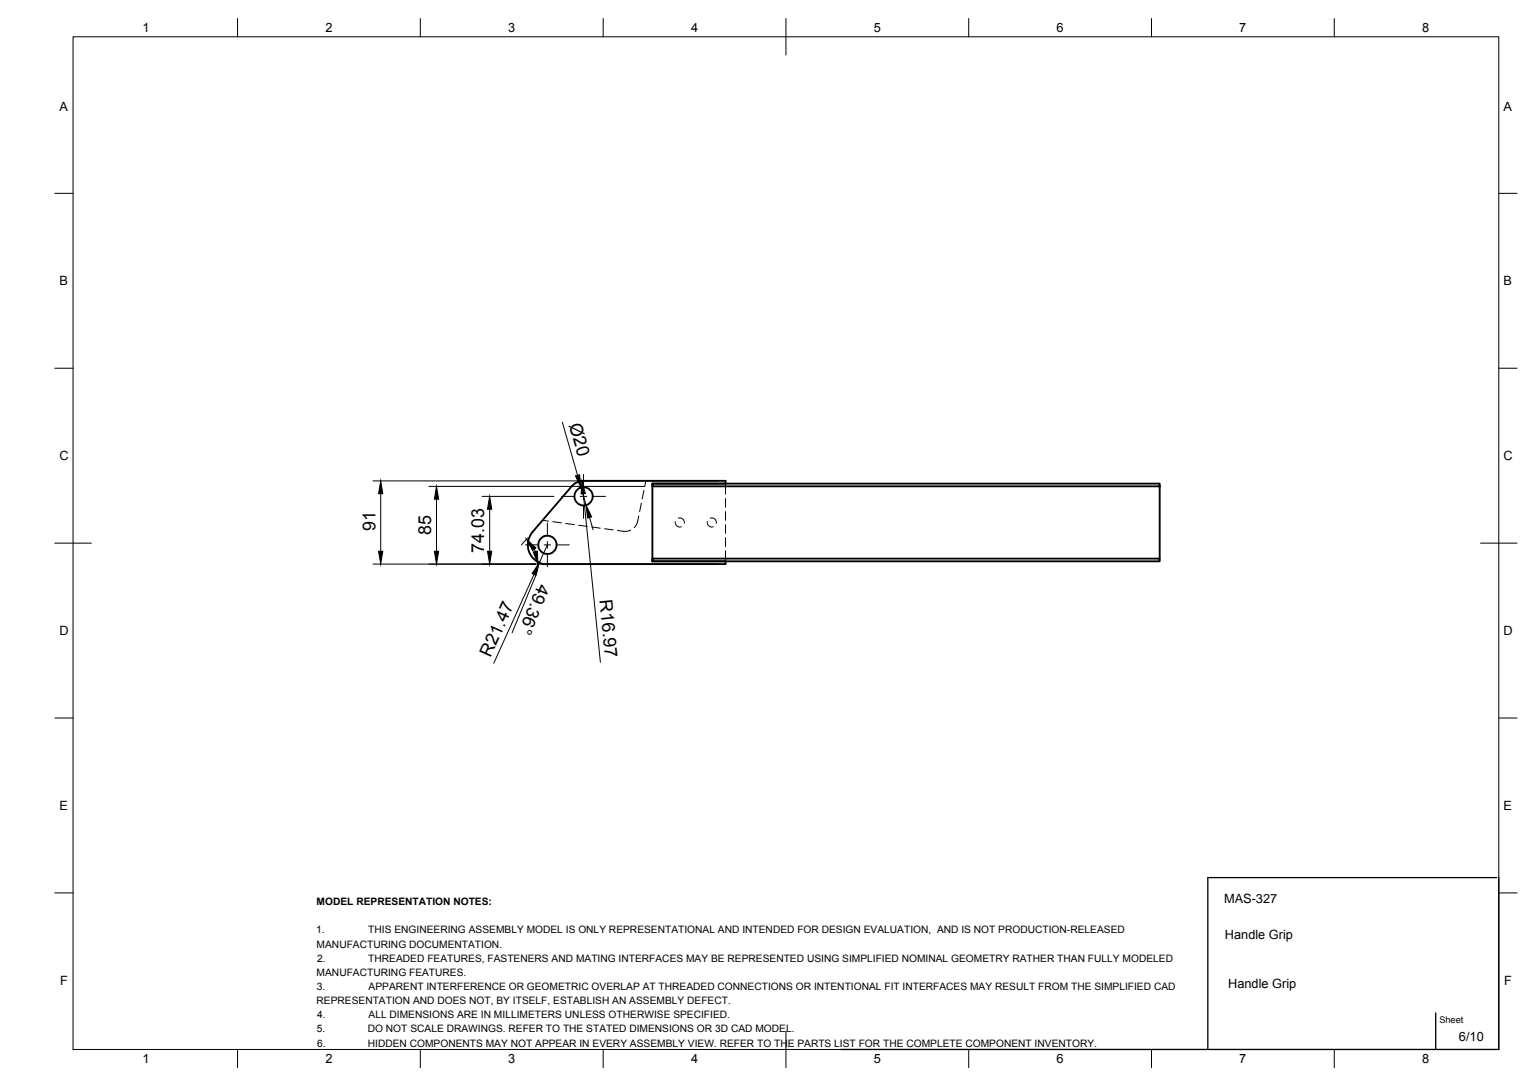
ISO-10303-21;
HEADER;
FILE_DESCRIPTION (('STEP AP214'),
    '1' );
FILE_NAME ('Handle Grip.step',
    '2026-10-06T22:16:42',
    ( '' ),
    ( '' ),
    'SwSTEP 2.0',
    'SolidWorks 2025',
    '' );
FILE_SCHEMA (( 'AUTOMOTIVE_DESIGN' ));
ENDSEC;

DATA;
#6=FILL_AREA_STYLE_COLOUR ( '', #17600 ) ;
#21=CARTESIAN_POINT ( 'NONE',  ( 157.5268905834513475, 193.0332408774651185, -5.999999999999950262 ) ) ;
#34=DIRECTION ( 'NONE',  ( 0.4874675571821265319, 0.8731411001063289490, -0.000000000000000000 ) ) ;
#90=LINE ( 'NONE', #6822, #7245 ) ;
#117=SURFACE_STYLE_FILL_AREA ( #8505 ) ;
#120=VERTEX_POINT ( 'NONE', #20084 ) ;
#156=CARTESIAN_POINT ( 'NONE',  ( 131.8222645499857322, 267.5435007770734046, -19.99999999999997868 ) ) ;
#159=CARTESIAN_POINT ( 'NONE',  ( 138.4260920561042667, 141.9264758756783351, 4.000000000000021316 ) ) ;
#165=CIRCLE ( 'NONE', #18804, 10.00000000000000888 ) ;
#169=ORIENTED_EDGE ( 'NONE', *, *, #12306, .F. ) ;
#196=AXIS2_PLACEMENT_3D ( 'NONE', #10385, #15763, #18755 ) ;
#214=CIRCLE ( 'NONE', #196, 21.47274291077713571 ) ;
#241=ADVANCED_FACE ( 'NONE', ( #14877 ), #10156, .F. ) ;
#244=AXIS2_PLACEMENT_3D ( 'NONE', #16241, #7884, #6214 ) ;
#255=VERTEX_POINT ( 'NONE', #6848 ) ;
#264=CARTESIAN_POINT ( 'NONE',  ( 109.8528842077358405, 344.7014318495014322, 4.000000000000003553 ) ) ;
#267=CARTESIAN_POINT ( 'NONE',  ( 109.8528842077358405, 344.7014318495014322, 272.0939500981630204 ) ) ;
#276=VECTOR ( 'NONE', #19328, 1000.000000000000000 ) ;
#283=MANIFOLD_SOLID_BREP ( 'Cut-Extrude11', #13403 ) ;
#304=CARTESIAN_POINT ( 'NONE',  ( 27.25521010731993243, 314.3399865783788414, -19.99999999999996092 ) ) ;
#348=LINE ( 'NONE', #7078, #20330 ) ;
#428=AXIS2_PLACEMENT_3D ( 'NONE', #10499, #19300, #5628 ) ;
#429=VECTOR ( 'NONE', #16565, 1000.000000000000000 ) ;
#443=ORIENTED_EDGE ( 'NONE', *, *, #13738, .F. ) ;
#452=DIRECTION ( 'NONE',  ( 0.000000000000000000, 0.000000000000000000, 1.000000000000000000 ) ) ;
#455=DIRECTION ( 'NONE',  ( 0.000000000000000000, 0.000000000000000000, 1.000000000000000000 ) ) ;
#474=VECTOR ( 'NONE', #11698, 1000.000000000000114 ) ;
#538=DIRECTION ( 'NONE',  ( 0.000000000000000000, 0.000000000000000000, 1.000000000000000000 ) ) ;
#586=ADVANCED_BREP_SHAPE_REPRESENTATION ( '', ( #14581, #283, #12657 ), #11603 ) ;
#604=ORIENTED_EDGE ( 'NONE', *, *, #3541, .T. ) ;
#632=VECTOR ( 'NONE', #4152, 1000.000000000000227 ) ;
#670=CARTESIAN_POINT ( 'NONE',  ( 111.4021762516569964, 137.5714195593754710, -19.99999999999997868 ) ) ;
#686=ORIENTED_EDGE ( 'NONE', *, *, #10694, .T. ) ;
#720=DIRECTION ( 'NONE',  ( 1.000000000000000000, 0.000000000000000000, 0.000000000000000000 ) ) ;
#758=DIRECTION ( 'NONE',  ( 1.000000000000000000, 0.000000000000000000, 0.000000000000000000 ) ) ;
#763=ADVANCED_FACE ( 'NONE', ( #12088 ), #11983, .F. ) ;
#857=( LENGTH_UNIT ( ) NAMED_UNIT ( * ) SI_UNIT ( .MILLI., .METRE. ) );
#899=ORIENTED_EDGE ( 'NONE', *, *, #19930, .T. ) ;
#900=VECTOR ( 'NONE', #10656, 1000.000000000000114 ) ;
#918=ORIENTED_EDGE ( 'NONE', *, *, #19173, .F. ) ;
#932=VECTOR ( 'NONE', #17024, 1000.000000000000227 ) ;
#984=CARTESIAN_POINT ( 'NONE',  ( 96.62434152388762243, 220.7958015105191976, 4.000000000000021316 ) ) ;
#988=EDGE_CURVE ( 'NONE', #1240, #17720, #90, .T. ) ;
#1025=ORIENTED_EDGE ( 'NONE', *, *, #8453, .F. ) ;
#1031=DIRECTION ( 'NONE',  ( -0.000000000000000000, -0.000000000000000000, -1.000000000000000000 ) ) ;
#1069=ADVANCED_FACE ( 'NONE', ( #8909 ), #19146, .F. ) ;
#1077=PLANE ( 'NONE',  #8255 ) ;
#1102=CARTESIAN_POINT ( 'NONE',  ( 109.8528842077358405, 344.7014318495014322, 4.000000000000003553 ) ) ;
#1138=VERTEX_POINT ( 'NONE', #9014 ) ;
#1157=SHAPE_DEFINITION_REPRESENTATION ( #11328, #17468 ) ;
#1165=ORIENTED_EDGE ( 'NONE', *, *, #14487, .T. ) ;
#1173=CARTESIAN_POINT ( 'NONE',  ( -56.84366818088135176, 789.5005544000622422, -3.999999999999996447 ) ) ;
#1239=EDGE_CURVE ( 'NONE', #13557, #19772, #12755, .T. ) ;
#1240=VERTEX_POINT ( 'NONE', #21355 ) ;
#1246=DIRECTION ( 'NONE',  ( -0.3450121214752274734, 0.9385982292947089300, 0.000000000000000000 ) ) ;
#1257=CYLINDRICAL_SURFACE ( 'NONE', #244, 5.000000000000004441 ) ;
#1258=LINE ( 'NONE', #14373, #6793 ) ;
#1303=VERTEX_POINT ( 'NONE', #3051 ) ;
#1312=DIRECTION ( 'NONE',  ( 0.000000000000000000, 0.000000000000000000, 1.000000000000000000 ) ) ;
#1315=DIRECTION ( 'NONE',  ( -0.3450121214752274179, 0.9385982292947088190, -0.000000000000000000 ) ) ;
#1334=VERTEX_POINT ( 'NONE', #19922 ) ;
#1335=ADVANCED_FACE ( 'NONE', ( #16484 ), #1400, .F. ) ;
#1357=ORIENTED_EDGE ( 'NONE', *, *, #19930, .F. ) ;
#1400=CYLINDRICAL_SURFACE ( 'NONE', #21320, 13.99821153497579651 ) ;
#1424=CARTESIAN_POINT ( 'NONE',  ( 147.5268905834513475, 193.0332408774651185, -5.999999999999976019 ) ) ;
#1451=CARTESIAN_POINT ( 'NONE',  ( 111.4021762516569964, 137.5714195593754710, -19.99999999999997868 ) ) ;
#1461=CARTESIAN_POINT ( 'NONE',  ( 77.34521997529867576, 314.8592298662555322, 272.0939500981630204 ) ) ;
#1503=ORIENTED_EDGE ( 'NONE', *, *, #17821, .F. ) ;
#1506=EDGE_CURVE ( 'NONE', #14220, #7040, #17142, .T. ) ;
#1536=FACE_OUTER_BOUND ( 'NONE', #21519, .T. ) ;
#1587=CARTESIAN_POINT ( 'NONE',  ( 24.43941541943582862, 313.3049502139530205, -19.99999999999997868 ) ) ;
#1590=PLANE ( 'NONE',  #20674 ) ;
#1634=EDGE_LOOP ( 'NONE', ( #6697, #6090, #8259, #12227, #10323, #12958 ) ) ;
#1642=ADVANCED_FACE ( 'NONE', ( #8572 ), #13730, .F. ) ;
#1643=CIRCLE ( 'NONE', #19950, 5.000000000000004441 ) ;
#1657=ORIENTED_EDGE ( 'NONE', *, *, #8443, .F. ) ;
#1725=ORIENTED_EDGE ( 'NONE', *, *, #10803, .F. ) ;
#1745=AXIS2_PLACEMENT_3D ( 'NONE', #8370, #15081, #21817 ) ;
#1778=ORIENTED_EDGE ( 'NONE', *, *, #3369, .T. ) ;
#1784=EDGE_CURVE ( 'NONE', #10393, #12279, #9220, .T. ) ;
#1786=DIRECTION ( 'NONE',  ( -0.000000000000000000, -0.000000000000000000, -1.000000000000000000 ) ) ;
#1826=DIRECTION ( 'NONE',  ( 1.000000000000000000, 0.000000000000000000, 0.000000000000000000 ) ) ;
#1838=CARTESIAN_POINT ( 'NONE',  ( 24.43941541943582862, 313.3049502139530205, 4.000000000000003553 ) ) ;
#1878=VERTEX_POINT ( 'NONE', #4903 ) ;
#1894=ORIENTED_EDGE ( 'NONE', *, *, #13085, .F. ) ;
#1917=CARTESIAN_POINT ( 'NONE',  ( 84.42064422693164261, 282.0082918409407284, 272.0939500981630204 ) ) ;
#1941=DIRECTION ( 'NONE',  ( -0.9385982292947088190, -0.3450121214752277510, 0.000000000000000000 ) ) ;
#1999=FACE_OUTER_BOUND ( 'NONE', #9695, .T. ) ;
#2013=ORIENTED_EDGE ( 'NONE', *, *, #20527, .F. ) ;
#2030=DIRECTION ( 'NONE',  ( -0.8510798296367590998, -0.5250363069212118372, 0.000000000000000000 ) ) ;
#2045=VERTEX_POINT ( 'NONE', #159 ) ;
#2047=ADVANCED_FACE ( 'NONE', ( #15478 ), #18460, .F. ) ;
#2048=CARTESIAN_POINT ( 'NONE',  ( 134.6380592378699532, 268.5785371414991687, -3.999999999999996447 ) ) ;
#2065=CYLINDRICAL_SURFACE ( 'NONE', #12749, 10.00000000000000888 ) ;
#2083=DIRECTION ( 'NONE',  ( -0.000000000000000000, -0.000000000000000000, -1.000000000000000000 ) ) ;
#2116=VERTEX_POINT ( 'NONE', #8653 ) ;
#2172=CIRCLE ( 'NONE', #428, 10.00000000000000888 ) ;
#2213=CARTESIAN_POINT ( 'NONE',  ( -136.6255475934131596, 760.1741454933652449, -19.99999999999996092 ) ) ;
#2221=ORIENTED_EDGE ( 'NONE', *, *, #4577, .F. ) ;
#2224=VERTEX_POINT ( 'NONE', #10307 ) ;
#2233=FACE_BOUND ( 'NONE', #12574, .T. ) ;
#2251=LINE ( 'NONE', #3913, #13441 ) ;
#2275=ADVANCED_FACE ( 'NONE', ( #20124 ), #17010, .F. ) ;
#2297=LINE ( 'NONE', #17284, #12378 ) ;
#2305=ORIENTED_EDGE ( 'NONE', *, *, #5717, .T. ) ;
#2349=EDGE_LOOP ( 'NONE', ( #3996, #12011, #2902, #18773, #11925, #10645 ) ) ;
#2356=ORIENTED_EDGE ( 'NONE', *, *, #5717, .F. ) ;
#2393=ORIENTED_EDGE ( 'NONE', *, *, #15930, .T. ) ;
#2399=EDGE_CURVE ( 'NONE', #9454, #17720, #16871, .T. ) ;
#2403=CARTESIAN_POINT ( 'NONE',  ( 0.000000000000000000, 0.000000000000000000, 0.000000000000000000 ) ) ;
#2417=VERTEX_POINT ( 'NONE', #18539 ) ;
#2424=DIRECTION ( 'NONE',  ( 0.9385982292947088190, 0.3450121214752278620, -0.000000000000000000 ) ) ;
#2436=EDGE_LOOP ( 'NONE', ( #12164, #19467, #16101, #7360, #18553, #14229, #20531, #9668 ) ) ;
#2476=EDGE_CURVE ( 'NONE', #1878, #10563, #4648, .T. ) ;
#2520=EDGE_CURVE ( 'NONE', #2224, #7555, #21637, .T. ) ;
#2547=ORIENTED_EDGE ( 'NONE', *, *, #1784, .F. ) ;
#2592=VERTEX_POINT ( 'NONE', #5201 ) ;
#2600=ORIENTED_EDGE ( 'NONE', *, *, #20829, .T. ) ;
#2619=CARTESIAN_POINT ( 'NONE',  ( 109.8528842077358405, 344.7014318495014322, -19.99999999999997868 ) ) ;
#2624=ORIENTED_EDGE ( 'NONE', *, *, #6281, .F. ) ;
#2626=VERTEX_POINT ( 'NONE', #13889 ) ;
#2628=CARTESIAN_POINT ( 'NONE',  ( 108.9927164799167372, 227.3511983043831037, -5.999999999999976019 ) ) ;
#2641=VECTOR ( 'NONE', #14185, 1000.000000000000227 ) ;
#2650=ORIENTED_EDGE ( 'NONE', *, *, #6268, .T. ) ;
#2672=AXIS2_PLACEMENT_3D ( 'NONE', #18216, #12932, #19656 ) ;
#2678=ORIENTED_EDGE ( 'NONE', *, *, #16774, .T. ) ;
#2682=EDGE_CURVE ( 'NONE', #13485, #15661, #214, .T. ) ;
#2686=CARTESIAN_POINT ( 'NONE',  ( 84.42064422693164261, 282.0082918409407284, 4.000000000000003553 ) ) ;
#2687=DIRECTION ( 'NONE',  ( 0.3450121214752276400, -0.9385982292947087080, 0.000000000000000000 ) ) ;
#2703=DIRECTION ( 'NONE',  ( -0.000000000000000000, -0.000000000000000000, 1.000000000000000000 ) ) ;
#2731=DIRECTION ( 'NONE',  ( 0.000000000000000000, 0.000000000000000000, 1.000000000000000000 ) ) ;
#2770=SURFACE_SIDE_STYLE ('',( #17858 ) ) ;
#2779=LINE ( 'NONE', #21415, #3675 ) ;
#2793=ORIENTED_EDGE ( 'NONE', *, *, #13155, .T. ) ;
#2794=CARTESIAN_POINT ( 'NONE',  ( 121.4021762516569964, 137.5714195593754710, 272.0939500981630204 ) ) ;
#2797=CARTESIAN_POINT ( 'NONE',  ( -136.6255475934131596, 760.1741454933652449, -19.99999999999996092 ) ) ;
#2828=DIRECTION ( 'NONE',  ( 1.000000000000000000, 0.000000000000000000, 0.000000000000000000 ) ) ;
#2831=DIRECTION ( 'NONE',  ( 1.000000000000000000, 0.000000000000000000, -1.723963091245776585E-16 ) ) ;
#2857=PLANE ( 'NONE',  #8341 ) ;
#2861=LINE ( 'NONE', #6061, #16612 ) ;
#2875=ADVANCED_FACE ( 'NONE', ( #11445 ), #11665, .F. ) ;
#2891=DIRECTION ( 'NONE',  ( -0.3450121214752278065, 0.9385982292947087080, -0.000000000000000000 ) ) ;
#2902=ORIENTED_EDGE ( 'NONE', *, *, #10237, .T. ) ;
#2904=LINE ( 'NONE', #16229, #19073 ) ;
#2945=EDGE_CURVE ( 'NONE', #7555, #1878, #9921, .T. ) ;
#2976=ORIENTED_EDGE ( 'NONE', *, *, #9209, .F. ) ;
#2987=ORIENTED_EDGE ( 'NONE', *, *, #15449, .T. ) ;
#2995=ADVANCED_FACE ( 'NONE', ( #14969 ), #21608, .F. ) ;
#2998=ADVANCED_FACE ( 'NONE', ( #1536 ), #13334, .F. ) ;
#3003=ORIENTED_EDGE ( 'NONE', *, *, #988, .F. ) ;
#3010=FACE_OUTER_BOUND ( 'NONE', #8960, .T. ) ;
#3011=PLANE ( 'NONE',  #9235 ) ;
#3051=CARTESIAN_POINT ( 'NONE',  ( 134.6380592378700101, 268.5785371414991687, -3.999999999999996447 ) ) ;
#3078=CARTESIAN_POINT ( 'NONE',  ( 111.4021762516569964, 137.5714195593754710, 272.0939500981630204 ) ) ;
#3126=EDGE_LOOP ( 'NONE', ( #4259, #8088, #5351, #15639 ) ) ;
#3135=DIRECTION ( 'NONE',  ( -0.9385982292947087080, -0.3450121214752278620, 0.000000000000000000 ) ) ;
#3154=ORIENTED_EDGE ( 'NONE', *, *, #5582, .F. ) ;
#3180=CARTESIAN_POINT ( 'NONE',  ( 96.62434152388763664, 220.7958015105191976, -5.999999999999976019 ) ) ;
#3233=VECTOR ( 'NONE', #34, 999.9999999999998863 ) ;
#3333=CIRCLE ( 'NONE', #20241, 10.00000000000000888 ) ;
#3336=DIRECTION ( 'NONE',  ( -0.4874675571821265319, -0.8731411001063289490, 0.000000000000000000 ) ) ;
#3355=ADVANCED_FACE ( 'NONE', ( #3010 ), #5985, .T. ) ;
#3358=CARTESIAN_POINT ( 'NONE',  ( 162.3411339277076308, 184.7625696037766261, 272.0939500981630204 ) ) ;
#3369=EDGE_CURVE ( 'NONE', #13485, #120, #16125, .T. ) ;
#3394=LINE ( 'NONE', #14169, #19787 ) ;
#3400=EDGE_CURVE ( 'NONE', #9553, #2626, #9376, .T. ) ;
#3475=CARTESIAN_POINT ( 'NONE',  ( 139.9279279298906147, 262.8829071470229906, 4.000000000000021316 ) ) ;
#3484=LINE ( 'NONE', #12162, #3741 ) ;
#3486=DIRECTION ( 'NONE',  ( 0.000000000000000000, 0.000000000000000000, 1.000000000000000000 ) ) ;
#3496=VECTOR ( 'NONE', #14530, 1000.000000000000000 ) ;
#3541=EDGE_CURVE ( 'NONE', #9751, #9805, #11486, .T. ) ;
#3590=CARTESIAN_POINT ( 'NONE',  ( -56.84366818088135176, 789.5005544000622422, -19.99999999999997868 ) ) ;
#3603=AXIS2_PLACEMENT_3D ( 'NONE', #9604, #13419, #11757 ) ;
#3617=LINE ( 'NONE', #304, #10490 ) ;
#3659=CARTESIAN_POINT ( 'NONE',  ( 134.6380592378700101, 268.5785371414991687, -19.99999999999997868 ) ) ;
#3675=VECTOR ( 'NONE', #19317, 1000.000000000000227 ) ;
#3680=EDGE_CURVE ( 'NONE', #17077, #17427, #12985, .T. ) ;
#3694=CARTESIAN_POINT ( 'NONE',  ( -136.6255475934131596, 760.1741454933652449, -3.999999999999980904 ) ) ;
#3704=FACE_OUTER_BOUND ( 'NONE', #19461, .T. ) ;
#3718=DIRECTION ( 'NONE',  ( -1.000000000000000000, 0.000000000000000000, 0.000000000000000000 ) ) ;
#3741=VECTOR ( 'NONE', #20560, 1000.000000000000000 ) ;
#3749=DIRECTION ( 'NONE',  ( -1.000000000000000000, 0.000000000000000000, 0.000000000000000000 ) ) ;
#3751=CARTESIAN_POINT ( 'NONE',  ( 84.42064422693164261, 282.0082918409407284, 272.0939500981630204 ) ) ;
#3766=CARTESIAN_POINT ( 'NONE',  ( 138.4260920561042667, 141.9264758756783351, -5.999999999999976019 ) ) ;
#3774=VECTOR ( 'NONE', #8378, 1000.000000000000000 ) ;
#3822=CARTESIAN_POINT ( 'NONE',  ( 131.8222645499855901, 267.5435007770738025, -6.999999999999995559 ) ) ;
#3835=EDGE_CURVE ( 'NONE', #11879, #1138, #3617, .T. ) ;
#3894=DIRECTION ( 'NONE',  ( 0.000000000000000000, 0.000000000000000000, 1.000000000000000000 ) ) ;
#3900=CARTESIAN_POINT ( 'NONE',  ( -56.84366818088135176, 789.5005544000622422, -19.99999999999997868 ) ) ;
#3913=CARTESIAN_POINT ( 'NONE',  ( -133.8097529055291943, 761.2091818577913500, -45.62971374797768220 ) ) ;
#3925=CARTESIAN_POINT ( 'NONE',  ( 162.3411339277076308, 184.7625696037766261, -19.99999999999997868 ) ) ;
#3933=ORIENTED_EDGE ( 'NONE', *, *, #13644, .T. ) ;
#3940=VECTOR ( 'NONE', #21428, 1000.000000000000227 ) ;
#3954=CIRCLE ( 'NONE', #12396, 5.000000000000004441 ) ;
#3986=DIRECTION ( 'NONE',  ( 1.723963091245776585E-16, 6.336983651701954299E-17, 1.000000000000000000 ) ) ;
#3996=ORIENTED_EDGE ( 'NONE', *, *, #11008, .T. ) ;
#4015=EDGE_LOOP ( 'NONE', ( #11908, #16204 ) ) ;
#4028=VECTOR ( 'NONE', #18971, 1000.000000000000000 ) ;
#4077=APPLICATION_CONTEXT ( 'automotive_design' ) ;
#4085=VECTOR ( 'NONE', #8189, 1000.000000000000114 ) ;
#4149=EDGE_CURVE ( 'NONE', #18306, #21732, #21020, .T. ) ;
#4152=DIRECTION ( 'NONE',  ( -0.9385982292947088190, -0.3450121214752274179, 2.040824802394967185E-16 ) ) ;
#4160=FACE_BOUND ( 'NONE', #14959, .T. ) ;
#4177=CARTESIAN_POINT ( 'NONE',  ( 134.6380592378700101, 268.5785371414991687, -19.99999999999997868 ) ) ;
#4227=EDGE_LOOP ( 'NONE', ( #4362, #2305, #1725, #918 ) ) ;
#4237=CARTESIAN_POINT ( 'NONE',  ( 139.9279279298906147, 262.8829071470229906, -5.999999999999976019 ) ) ;
#4259=ORIENTED_EDGE ( 'NONE', *, *, #4577, .T. ) ;
#4313=FACE_BOUND ( 'NONE', #6310, .T. ) ;
#4362=ORIENTED_EDGE ( 'NONE', *, *, #4637, .T. ) ;
#4382=EDGE_CURVE ( 'NONE', #1334, #1240, #7899, .T. ) ;
#4408=EDGE_CURVE ( 'NONE', #10633, #13533, #16149, .T. ) ;
#4413=FILL_AREA_STYLE ('',( #19520 ) ) ;
#4416=LINE ( 'NONE', #13242, #10438 ) ;
#4431=AXIS2_PLACEMENT_3D ( 'NONE', #19436, #1246, #11054 ) ;
#4434=VECTOR ( 'NONE', #16810, 1000.000000000000114 ) ;
#4495=DIRECTION ( 'NONE',  ( 1.723963091245776585E-16, 6.336983651701954299E-17, 1.000000000000000000 ) ) ;
#4527=( NAMED_UNIT ( * ) PLANE_ANGLE_UNIT ( ) SI_UNIT ( $, .RADIAN. ) );
#4561=DIRECTION ( 'NONE',  ( 1.000000000000000000, 0.000000000000000000, 0.000000000000000000 ) ) ;
#4577=EDGE_CURVE ( 'NONE', #17533, #10563, #8559, .T. ) ;
#4589=( NAMED_UNIT ( * ) PLANE_ANGLE_UNIT ( ) SI_UNIT ( $, .RADIAN. ) );
#4617=CARTESIAN_POINT ( 'NONE',  ( 54.85617982533816672, 239.2521282348021714, -19.99999999999996092 ) ) ;
#4618=FACE_OUTER_BOUND ( 'NONE', #16919, .T. ) ;
#4637=EDGE_CURVE ( 'NONE', #9746, #9069, #4827, .T. ) ;
#4648=LINE ( 'NONE', #11367, #4085 ) ;
#4653=CARTESIAN_POINT ( 'NONE',  ( 96.62434152388763664, 220.7958015105191976, 4.000000000000021316 ) ) ;
#4656=( GEOMETRIC_REPRESENTATION_CONTEXT ( 3 ) GLOBAL_UNCERTAINTY_ASSIGNED_CONTEXT ( ( #17219 ) ) GLOBAL_UNIT_ASSIGNED_CONTEXT ( ( #19634, #4527, #9617 ) ) REPRESENTATION_CONTEXT ( 'NONE', 'WORKASPACE' ) );
#4665=CARTESIAN_POINT ( 'NONE',  ( 93.25569916848381524, 126.0916958004080755, -19.99999999999997868 ) ) ;
#4668=ADVANCED_FACE ( 'NONE', ( #13609 ), #20347, .F. ) ;
#4692=ORIENTED_EDGE ( 'NONE', *, *, #4769, .T. ) ;
#4725=DIRECTION ( 'NONE',  ( -1.723963091245776092E-16, -6.336983651701951834E-17, -1.000000000000000000 ) ) ;
#4769=EDGE_CURVE ( 'NONE', #1878, #255, #12607, .T. ) ;
#4773=VECTOR ( 'NONE', #1786, 1000.000000000000000 ) ;
#4775=VERTEX_POINT ( 'NONE', #9307 ) ;
#4780=VECTOR ( 'NONE', #18040, 1000.000000000000000 ) ;
#4827=CIRCLE ( 'NONE', #16087, 10.00000000000000888 ) ;
#4839=LINE ( 'NONE', #16404, #18906 ) ;
#4862=VERTEX_POINT ( 'NONE', #13708 ) ;
#4902=CARTESIAN_POINT ( 'NONE',  ( 27.25521010731993243, 314.3399865783788414, -19.99999999999996092 ) ) ;
#4903=CARTESIAN_POINT ( 'NONE',  ( 134.6380592378699532, 268.5785371414991687, -19.99999999999997868 ) ) ;
#4913=ORIENTED_EDGE ( 'NONE', *, *, #6688, .F. ) ;
#4922=AXIS2_PLACEMENT_3D ( 'NONE', #10433, #10650, #19233 ) ;
#4959=CARTESIAN_POINT ( 'NONE',  ( 137.5268905834513191, 193.0332408774651185, 272.0939500981630204 ) ) ;
#5018=DIRECTION ( 'NONE',  ( -0.9385982292947088190, -0.3450121214752277510, 0.000000000000000000 ) ) ;
#5027=CARTESIAN_POINT ( 'NONE',  ( 107.0370895198517189, 343.6663954850758955, -19.99999999999997868 ) ) ;
#5046=PLANE ( 'NONE',  #3603 ) ;
#5057=ORIENTED_EDGE ( 'NONE', *, *, #13409, .T. ) ;
#5066=DIRECTION ( 'NONE',  ( -0.000000000000000000, -0.000000000000000000, -1.000000000000000000 ) ) ;
#5107=CARTESIAN_POINT ( 'NONE',  ( -56.84366818088135176, 789.5005544000622422, -3.999999999999996447 ) ) ;
#5138=VERTEX_POINT ( 'NONE', #7655 ) ;
#5143=CARTESIAN_POINT ( 'NONE',  ( 24.43941541943582862, 313.3049502139530205, 4.000000000000003553 ) ) ;
#5157=DIRECTION ( 'NONE',  ( -0.3450121214752276955, 0.9385982292947087080, -0.000000000000000000 ) ) ;
#5177=EDGE_CURVE ( 'NONE', #20168, #2045, #17869, .T. ) ;
#5188=AXIS2_PLACEMENT_3D ( 'NONE', #9596, #16187, #12564 ) ;
#5201=CARTESIAN_POINT ( 'NONE',  ( -136.6255475934131596, 760.1741454933652449, -3.999999999999980904 ) ) ;
#5223=ORIENTED_EDGE ( 'NONE', *, *, #17821, .T. ) ;
#5255=LINE ( 'NONE', #5566, #8719 ) ;
#5292=SURFACE_STYLE_USAGE ( .BOTH. , #18633 ) ;
#5294=EDGE_CURVE ( 'NONE', #2224, #1138, #12811, .T. ) ;
#5299=ORIENTED_EDGE ( 'NONE', *, *, #4637, .F. ) ;
#5314=FACE_OUTER_BOUND ( 'NONE', #21176, .T. ) ;
#5351=ORIENTED_EDGE ( 'NONE', *, *, #2945, .F. ) ;
#5356=CARTESIAN_POINT ( 'NONE',  ( 24.43941541943582862, 313.3049502139530205, -19.99999999999997868 ) ) ;
#5368=EDGE_CURVE ( 'NONE', #16231, #17982, #15120, .T. ) ;
#5387=LINE ( 'NONE', #10360, #15011 ) ;
#5445=DIRECTION ( 'NONE',  ( 0.3450121214752278065, -0.9385982292947087080, -0.000000000000000000 ) ) ;
#5566=CARTESIAN_POINT ( 'NONE',  ( -56.84366818088135176, 789.5005544000622422, -3.999999999999996447 ) ) ;
#5574=VERTEX_POINT ( 'NONE', #19191 ) ;
#5582=EDGE_CURVE ( 'NONE', #13398, #4862, #20344, .T. ) ;
#5628=DIRECTION ( 'NONE',  ( 1.000000000000000000, 0.000000000000000000, 0.000000000000000000 ) ) ;
#5632=ORIENTED_EDGE ( 'NONE', *, *, #6281, .T. ) ;
#5634=AXIS2_PLACEMENT_3D ( 'NONE', #3751, #12113, #15102 ) ;
#5684=ADVANCED_FACE ( 'NONE', ( #14543 ), #5046, .F. ) ;
#5700=PLANE ( 'NONE',  #21103 ) ;
#5717=EDGE_CURVE ( 'NONE', #9069, #5138, #2861, .T. ) ;
#5736=DIRECTION ( 'NONE',  ( 1.000000000000000000, 0.000000000000000000, -1.734723475976805615E-16 ) ) ;
#5801=AXIS2_PLACEMENT_3D ( 'NONE', #20467, #18807, #10442 ) ;
#5841=DIRECTION ( 'NONE',  ( 1.000000000000000000, 0.000000000000000000, -1.734723475976805615E-16 ) ) ;
#5856=VECTOR ( 'NONE', #16236, 1000.000000000000227 ) ;
#5875=EDGE_LOOP ( 'NONE', ( #15537, #17424, #3154, #11551 ) ) ;
#5910=ORIENTED_EDGE ( 'NONE', *, *, #20563, .T. ) ;
#5945=AXIS2_PLACEMENT_3D ( 'NONE', #2628, #13908, #15568 ) ;
#5953=ADVANCED_FACE ( 'NONE', ( #7031 ), #2065, .F. ) ;
#5960=EDGE_CURVE ( 'NONE', #10863, #7143, #3394, .T. ) ;
#5985=PLANE ( 'NONE',  #4431 ) ;
#6018=CARTESIAN_POINT ( 'NONE',  ( 107.0370895198517189, 343.6663954850758955, -3.999999999999996447 ) ) ;
#6034=APPLICATION_CONTEXT ( 'automotive_design' ) ;
#6039=VECTOR ( 'NONE', #15498, 1000.000000000000227 ) ;
#6048=AXIS2_PLACEMENT_3D ( 'NONE', #18233, #13494, #3135 ) ;
#6061=CARTESIAN_POINT ( 'NONE',  ( 157.5268905834513475, 193.0332408774651185, 272.0939500981630204 ) ) ;
#6075=ORIENTED_EDGE ( 'NONE', *, *, #17476, .T. ) ;
#6085=ORIENTED_EDGE ( 'NONE', *, *, #10169, .F. ) ;
#6090=ORIENTED_EDGE ( 'NONE', *, *, #4408, .F. ) ;
#6140=CARTESIAN_POINT ( 'NONE',  ( 138.4260920561042667, 141.9264758756783351, -5.999999999999976019 ) ) ;
#6214=DIRECTION ( 'NONE',  ( -1.000000000000000000, 0.000000000000000000, 0.000000000000000000 ) ) ;
#6254=DIRECTION ( 'NONE',  ( 0.4874675571821264763, 0.8731411001063288380, 0.000000000000000000 ) ) ;
#6255=LINE ( 'NONE', #17714, #19428 ) ;
#6268=EDGE_CURVE ( 'NONE', #17720, #10563, #10329, .T. ) ;
#6274=CYLINDRICAL_SURFACE ( 'NONE', #9672, 16.96660865288809816 ) ;
#6281=EDGE_CURVE ( 'NONE', #8122, #12991, #10294, .T. ) ;
#6310=EDGE_LOOP ( 'NONE', ( #2393, #604 ) ) ;
#6320=VERTEX_POINT ( 'NONE', #5143 ) ;
#6347=ORIENTED_EDGE ( 'NONE', *, *, #2520, .F. ) ;
#6383=CARTESIAN_POINT ( 'NONE',  ( -136.6255475934131596, 760.1741454933652449, -3.999999999999980904 ) ) ;
#6384=LINE ( 'NONE', #4617, #15109 ) ;
#6401=ORIENTED_EDGE ( 'NONE', *, *, #2476, .T. ) ;
#6419=PRODUCT ( 'Handle Grip', 'Handle Grip', '', ( #19556 ) ) ;
#6420=COLOUR_RGB ( '', 0.72549020, 0.75294118, 0.79215686) ;
#6454=DIRECTION ( 'NONE',  ( -0.000000000000000000, -0.000000000000000000, -1.000000000000000000 ) ) ;
#6485=ORIENTED_EDGE ( 'NONE', *, *, #3835, .T. ) ;
#6545=AXIS2_PLACEMENT_3D ( 'NONE', #267, #5018, #8439 ) ;
#6548=EDGE_LOOP ( 'NONE', ( #17582, #11767, #6991, #9856 ) ) ;
#6556=VECTOR ( 'NONE', #5445, 1000.000000000000114 ) ;
#6601=CARTESIAN_POINT ( 'NONE',  ( 72.34521997529867576, 314.8592298662555322, 272.0939500981630204 ) ) ;
#6603=ORIENTED_EDGE ( 'NONE', *, *, #13085, .T. ) ;
#6610=AXIS2_PLACEMENT_3D ( 'NONE', #14704, #14590, #21667 ) ;
#6634=AXIS2_PLACEMENT_3D ( 'NONE', #4237, #21003, #8892 ) ;
#6655=PRODUCT_DEFINITION_CONTEXT ( 'detailed design', #4077, 'design' ) ;
#6688=EDGE_CURVE ( 'NONE', #6320, #13485, #1258, .T. ) ;
#6697=ORIENTED_EDGE ( 'NONE', *, *, #18056, .F. ) ;
#6743=ORIENTED_EDGE ( 'NONE', *, *, #7316, .F. ) ;
#6761=CARTESIAN_POINT ( 'NONE',  ( 54.85617982533818804, 239.2521282348021714, -19.99999999999996092 ) ) ;
#6782=CARTESIAN_POINT ( 'NONE',  ( 93.25569916848381524, 126.0916958004080755, 272.0939500981630204 ) ) ;
#6793=VECTOR ( 'NONE', #2687, 1000.000000000000227 ) ;
#6814=CARTESIAN_POINT ( 'NONE',  ( -133.8097529055291943, 761.2091818577913500, -6.999999999999982236 ) ) ;
#6822=CARTESIAN_POINT ( 'NONE',  ( 109.8528842077358405, 344.7014318495014322, -19.99999999999997868 ) ) ;
#6838=DIRECTION ( 'NONE',  ( 0.000000000000000000, 0.000000000000000000, 1.000000000000000000 ) ) ;
#6848=CARTESIAN_POINT ( 'NONE',  ( 54.85617982533816672, 239.2521282348021714, -19.99999999999996092 ) ) ;
#6884=VECTOR ( 'NONE', #10224, 1000.000000000000227 ) ;
#6904=DIRECTION ( 'NONE',  ( -0.3450121214752274179, 0.9385982292947088190, -7.395570986446985676E-32 ) ) ;
#6913=DIRECTION ( 'NONE',  ( 1.000000000000000000, 0.000000000000000000, 0.000000000000000000 ) ) ;
#6931=VECTOR ( 'NONE', #7320, 1000.000000000000000 ) ;
#6991=ORIENTED_EDGE ( 'NONE', *, *, #8037, .T. ) ;
#7018=VERTEX_POINT ( 'NONE', #11836 ) ;
#7031=FACE_OUTER_BOUND ( 'NONE', #4227, .T. ) ;
#7040=VERTEX_POINT ( 'NONE', #15256 ) ;
#7050=DIRECTION ( 'NONE',  ( 0.000000000000000000, 0.000000000000000000, 1.000000000000000000 ) ) ;
#7062=( NAMED_UNIT ( * ) SI_UNIT ( $, .STERADIAN. ) SOLID_ANGLE_UNIT ( ) );
#7078=CARTESIAN_POINT ( 'NONE',  ( 24.43941541943582862, 313.3049502139530205, 272.0939500981630204 ) ) ;
#7084=CARTESIAN_POINT ( 'NONE',  ( 162.3411339277076308, 184.7625696037766261, 272.0939500981630204 ) ) ;
#7097=ORIENTED_EDGE ( 'NONE', *, *, #20930, .T. ) ;
#7100=DIRECTION ( 'NONE',  ( 0.9385982292947088190, 0.3450121214752276955, -0.000000000000000000 ) ) ;
#7143=VERTEX_POINT ( 'NONE', #21664 ) ;
#7144=DIRECTION ( 'NONE',  ( 0.000000000000000000, 0.000000000000000000, 1.000000000000000000 ) ) ;
#7149=ORIENTED_EDGE ( 'NONE', *, *, #19173, .T. ) ;
#7169=DIRECTION ( 'NONE',  ( -0.9385982292947088190, -0.3450121214752274179, 2.040824802394967185E-16 ) ) ;
#7234=ORIENTED_EDGE ( 'NONE', *, *, #21469, .F. ) ;
#7245=VECTOR ( 'NONE', #5157, 1000.000000000000227 ) ;
#7279=AXIS2_PLACEMENT_3D ( 'NONE', #21086, #8862, #14019 ) ;
#7291=VECTOR ( 'NONE', #1941, 999.9999999999998863 ) ;
#7298=DIRECTION ( 'NONE',  ( -0.3450121214752275844, 0.9385982292947088190, 0.000000000000000000 ) ) ;
#7316=EDGE_CURVE ( 'NONE', #255, #11879, #6384, .T. ) ;
#7320=DIRECTION ( 'NONE',  ( 0.000000000000000000, 0.000000000000000000, -1.000000000000000000 ) ) ;
#7330=ORIENTED_EDGE ( 'NONE', *, *, #20404, .F. ) ;
#7360=ORIENTED_EDGE ( 'NONE', *, *, #20527, .T. ) ;
#7403=DIRECTION ( 'NONE',  ( -0.3450121214752278065, 0.9385982292947087080, 0.000000000000000000 ) ) ;
#7411=ORIENTED_EDGE ( 'NONE', *, *, #20563, .F. ) ;
#7420=ORIENTED_EDGE ( 'NONE', *, *, #2520, .T. ) ;
#7444=ORIENTED_EDGE ( 'NONE', *, *, #15000, .T. ) ;
#7463=EDGE_LOOP ( 'NONE', ( #6485, #8526, #443, #18927 ) ) ;
#7473=EDGE_LOOP ( 'NONE', ( #8482, #10075, #9524, #20401 ) ) ;
#7483=CARTESIAN_POINT ( 'NONE',  ( 57.67197451322198276, 240.2871645992281628, -6.999999999999982236 ) ) ;
#7519=EDGE_LOOP ( 'NONE', ( #4692, #16423, #7420, #12447 ) ) ;
#7555=VERTEX_POINT ( 'NONE', #8822 ) ;
#7621=VECTOR ( 'NONE', #1031, 1000.000000000000000 ) ;
#7644=EDGE_CURVE ( 'NONE', #9069, #9746, #3333, .T. ) ;
#7655=CARTESIAN_POINT ( 'NONE',  ( 157.5268905834513475, 193.0332408774651185, -19.99999999999997868 ) ) ;
#7706=DIRECTION ( 'NONE',  ( 1.723963091245776585E-16, 6.336983651701954299E-17, 1.000000000000000000 ) ) ;
#7773=ORIENTED_EDGE ( 'NONE', *, *, #8895, .F. ) ;
#7775=CARTESIAN_POINT ( 'NONE',  ( -136.6255475934131596, 760.1741454933652449, -3.999999999999980904 ) ) ;
#7824=ORIENTED_EDGE ( 'NONE', *, *, #10237, .F. ) ;
#7826=LINE ( 'NONE', #16396, #3496 ) ;
#7850=EDGE_CURVE ( 'NONE', #19966, #4862, #18268, .T. ) ;
#7882=LINE ( 'NONE', #7775, #5856 ) ;
#7884=DIRECTION ( 'NONE',  ( -0.000000000000000000, -0.000000000000000000, -1.000000000000000000 ) ) ;
#7888=CYLINDRICAL_SURFACE ( 'NONE', #6610, 21.47274291077713571 ) ;
#7899=LINE ( 'NONE', #12846, #17502 ) ;
#7914=DIRECTION ( 'NONE',  ( -0.000000000000000000, -0.000000000000000000, 1.000000000000000000 ) ) ;
#8037=EDGE_CURVE ( 'NONE', #8122, #21618, #11078, .T. ) ;
#8047=DIRECTION ( 'NONE',  ( 1.000000000000000000, 0.000000000000000000, 0.000000000000000000 ) ) ;
#8067=ORIENTED_EDGE ( 'NONE', *, *, #9771, .F. ) ;
#8088=ORIENTED_EDGE ( 'NONE', *, *, #2476, .F. ) ;
#8122=VERTEX_POINT ( 'NONE', #19460 ) ;
#8176=VERTEX_POINT ( 'NONE', #14171 ) ;
#8189=DIRECTION ( 'NONE',  ( -0.3450121214752278065, 0.9385982292947087080, -0.000000000000000000 ) ) ;
#8193=DIRECTION ( 'NONE',  ( 0.4683024526015100442, -0.8835682276357669229, 0.000000000000000000 ) ) ;
#8226=ORIENTED_EDGE ( 'NONE', *, *, #17669, .F. ) ;
#8255=AXIS2_PLACEMENT_3D ( 'NONE', #16276, #7706, #2831 ) ;
#8257=ADVANCED_FACE ( 'NONE', ( #14714 ), #15043, .F. ) ;
#8259=ORIENTED_EDGE ( 'NONE', *, *, #11008, .F. ) ;
#8287=ORIENTED_EDGE ( 'NONE', *, *, #9209, .T. ) ;
#8318=DIRECTION ( 'NONE',  ( -0.9385982292947087080, -0.3450121214752276955, -0.000000000000000000 ) ) ;
#8323=FACE_OUTER_BOUND ( 'NONE', #7519, .T. ) ;
#8341=AXIS2_PLACEMENT_3D ( 'NONE', #10816, #21167, #15973 ) ;
#8370=CARTESIAN_POINT ( 'NONE',  ( 72.34521997529867576, 314.8592298662555322, -4.000000000000003553 ) ) ;
#8378=DIRECTION ( 'NONE',  ( 0.000000000000000000, 0.000000000000000000, -1.000000000000000000 ) ) ;
#8393=CIRCLE ( 'NONE', #21765, 21.47274291077713571 ) ;
#8437=CARTESIAN_POINT ( 'NONE',  ( 162.3411339277076308, 184.7625696037766261, -19.99999999999997868 ) ) ;
#8439=DIRECTION ( 'NONE',  ( 0.3450121214752276955, -0.9385982292947087080, 0.000000000000000000 ) ) ;
#8443=EDGE_CURVE ( 'NONE', #2592, #20087, #9876, .T. ) ;
#8444=VECTOR ( 'NONE', #14827, 1000.000000000000000 ) ;
#8453=EDGE_CURVE ( 'NONE', #15661, #10393, #3484, .T. ) ;
#8482=ORIENTED_EDGE ( 'NONE', *, *, #14487, .F. ) ;
#8505=FILL_AREA_STYLE ('',( #6 ) ) ;
#8521=LINE ( 'NONE', #6761, #9991 ) ;
#8526=ORIENTED_EDGE ( 'NONE', *, *, #5294, .F. ) ;
#8552=DIRECTION ( 'NONE',  ( 0.000000000000000000, 0.000000000000000000, -1.000000000000000000 ) ) ;
#8559=LINE ( 'NONE', #5027, #14343 ) ;
#8572=FACE_OUTER_BOUND ( 'NONE', #16584, .T. ) ;
#8620=CIRCLE ( 'NONE', #18104, 13.99821153497579651 ) ;
#8644=PLANE ( 'NONE',  #14648 ) ;
#8653=CARTESIAN_POINT ( 'NONE',  ( 79.42064422693164261, 282.0082918409407284, 4.000000000000003553 ) ) ;
#8667=LINE ( 'NONE', #2048, #4434 ) ;
#8672=AXIS2_PLACEMENT_3D ( 'NONE', #3078, #9814, #20070 ) ;
#8673=CARTESIAN_POINT ( 'NONE',  ( 108.9927164799167372, 227.3511983043831037, -5.999999999999976019 ) ) ;
#8701=CIRCLE ( 'NONE', #5188, 5.000000000000004441 ) ;
#8719=VECTOR ( 'NONE', #19026, 1000.000000000000114 ) ;
#8721=PLANE ( 'NONE',  #13104 ) ;
#8738=CARTESIAN_POINT ( 'NONE',  ( 57.67197451322208934, 240.2871645992278218, 0.000000000000000000 ) ) ;
#8776=ORIENTED_EDGE ( 'NONE', *, *, #8037, .F. ) ;
#8822=CARTESIAN_POINT ( 'NONE',  ( 134.6380592378699532, 268.5785371414991687, -3.999999999999996447 ) ) ;
#8827=( LENGTH_UNIT ( ) NAMED_UNIT ( * ) SI_UNIT ( .MILLI., .METRE. ) );
#8830=EDGE_LOOP ( 'NONE', ( #5910, #16306 ) ) ;
#8858=ORIENTED_EDGE ( 'NONE', *, *, #9429, .F. ) ;
#8862=DIRECTION ( 'NONE',  ( 0.000000000000000000, 0.000000000000000000, 1.000000000000000000 ) ) ;
#8883=ORIENTED_EDGE ( 'NONE', *, *, #13409, .F. ) ;
#8887=EDGE_CURVE ( 'NONE', #7018, #20087, #8521, .T. ) ;
#8892=DIRECTION ( 'NONE',  ( -0.8510798296367592108, -0.5250363069212118372, 0.000000000000000000 ) ) ;
#8895=EDGE_CURVE ( 'NONE', #10633, #10863, #18320, .T. ) ;
#8909=FACE_OUTER_BOUND ( 'NONE', #2436, .T. ) ;
#8945=LINE ( 'NONE', #3766, #4028 ) ;
#8960=EDGE_LOOP ( 'NONE', ( #17910, #9586, #14470, #6603, #3933, #13236, #15986, #20451 ) ) ;
#8966=LINE ( 'NONE', #15672, #6931 ) ;
#8989=EDGE_LOOP ( 'NONE', ( #2624, #12791 ) ) ;
#9014=CARTESIAN_POINT ( 'NONE',  ( 27.25521010731993243, 314.3399865783788414, -3.999999999999980904 ) ) ;
#9039=DIRECTION ( 'NONE',  ( 0.4683024526015100442, -0.8835682276357669229, 0.000000000000000000 ) ) ;
#9069=VERTEX_POINT ( 'NONE', #21 ) ;
#9149=CARTESIAN_POINT ( 'NONE',  ( 107.0370895198517189, 343.6663954850758955, -3.999999999999996447 ) ) ;
#9183=ORIENTED_EDGE ( 'NONE', *, *, #18437, .F. ) ;
#9209=EDGE_CURVE ( 'NONE', #120, #10393, #8393, .T. ) ;
#9220=LINE ( 'NONE', #3925, #900 ) ;
#9235=AXIS2_PLACEMENT_3D ( 'NONE', #5107, #16669, #13482 ) ;
#9241=FACE_BOUND ( 'NONE', #8989, .T. ) ;
#9247=VECTOR ( 'NONE', #8552, 1000.000000000000000 ) ;
#9307=CARTESIAN_POINT ( 'NONE',  ( -136.6255475934131596, 760.1741454933652449, -19.99999999999996092 ) ) ;
#9320=ADVANCED_FACE ( 'NONE', ( #17951 ), #2857, .F. ) ;
#9374=CARTESIAN_POINT ( 'NONE',  ( 134.6380592378699532, 268.5785371414991687, -19.99999999999997868 ) ) ;
#9376=CIRCLE ( 'NONE', #2672, 10.00000000000000888 ) ;
#9378=DIRECTION ( 'NONE',  ( 0.000000000000000000, 0.000000000000000000, 1.000000000000000000 ) ) ;
#9418=CARTESIAN_POINT ( 'NONE',  ( 79.42064422693164261, 282.0082918409407284, 272.0939500981630204 ) ) ;
#9429=EDGE_CURVE ( 'NONE', #2116, #19966, #1643, .T. ) ;
#9431=DIRECTION ( 'NONE',  ( 0.000000000000000000, 0.000000000000000000, 1.000000000000000000 ) ) ;
#9448=EDGE_LOOP ( 'NONE', ( #5632, #2987, #7411, #8776 ) ) ;
#9454=VERTEX_POINT ( 'NONE', #1102 ) ;
#9461=EDGE_CURVE ( 'NONE', #8176, #21618, #14298, .T. ) ;
#9493=DIRECTION ( 'NONE',  ( 1.723963091245776585E-16, 6.336983651701954299E-17, 1.000000000000000000 ) ) ;
#9510=SURFACE_STYLE_USAGE ( .BOTH. , #2770 ) ;
#9524=ORIENTED_EDGE ( 'NONE', *, *, #20404, .T. ) ;
#9532=DIRECTION ( 'NONE',  ( -0.000000000000000000, -0.000000000000000000, -1.000000000000000000 ) ) ;
#9535=DIRECTION ( 'NONE',  ( -0.000000000000000000, -0.000000000000000000, -1.000000000000000000 ) ) ;
#9540=FACE_OUTER_BOUND ( 'NONE', #6548, .T. ) ;
#9553=VERTEX_POINT ( 'NONE', #13220 ) ;
#9576=AXIS2_PLACEMENT_3D ( 'NONE', #7084, #18546, #3336 ) ;
#9578=VECTOR ( 'NONE', #7169, 1000.000000000000227 ) ;
#9586=ORIENTED_EDGE ( 'NONE', *, *, #18437, .T. ) ;
#9596=CARTESIAN_POINT ( 'NONE',  ( 72.34521997529867576, 314.8592298662555322, 4.000000000000003553 ) ) ;
#9599=DIRECTION ( 'NONE',  ( -0.000000000000000000, -0.000000000000000000, -1.000000000000000000 ) ) ;
#9604=CARTESIAN_POINT ( 'NONE',  ( 57.67197451322198276, 240.2871645992281628, -45.62971374797768220 ) ) ;
#9617=( NAMED_UNIT ( * ) SI_UNIT ( $, .STERADIAN. ) SOLID_ANGLE_UNIT ( ) );
#9631=ORIENTED_EDGE ( 'NONE', *, *, #5582, .T. ) ;
#9662=ORIENTED_EDGE ( 'NONE', *, *, #5177, .T. ) ;
#9668=ORIENTED_EDGE ( 'NONE', *, *, #8887, .F. ) ;
#9671=LINE ( 'NONE', #6018, #10541 ) ;
#9672=AXIS2_PLACEMENT_3D ( 'NONE', #19503, #9599, #19396 ) ;
#9695=EDGE_LOOP ( 'NONE', ( #12135, #1657, #8067, #2793 ) ) ;
#9704=CARTESIAN_POINT ( 'NONE',  ( 134.6380592378700101, 268.5785371414991687, -3.999999999999996447 ) ) ;
#9721=ORIENTED_EDGE ( 'NONE', *, *, #13644, .F. ) ;
#9746=VERTEX_POINT ( 'NONE', #19055 ) ;
#9751=VERTEX_POINT ( 'NONE', #13865 ) ;
#9771=EDGE_CURVE ( 'NONE', #4775, #2592, #5387, .T. ) ;
#9773=ORIENTED_EDGE ( 'NONE', *, *, #18784, .F. ) ;
#9805=VERTEX_POINT ( 'NONE', #18948 ) ;
#9814=DIRECTION ( 'NONE',  ( -0.000000000000000000, -0.000000000000000000, -1.000000000000000000 ) ) ;
#9835=AXIS2_PLACEMENT_3D ( 'NONE', #11221, #19827, #21488 ) ;
#9856=ORIENTED_EDGE ( 'NONE', *, *, #9461, .F. ) ;
#9876=LINE ( 'NONE', #3694, #6556 ) ;
#9909=DIRECTION ( 'NONE',  ( 0.4683024526015100442, -0.8835682276357670339, 0.000000000000000000 ) ) ;
#9921=LINE ( 'NONE', #18508, #16407 ) ;
#9944=EDGE_LOOP ( 'NONE', ( #7097, #15565, #6347, #19492 ) ) ;
#9951=DIRECTION ( 'NONE',  ( 0.9385982292947087080, 0.3450121214752278620, -1.836742322155470738E-16 ) ) ;
#9971=ORIENTED_EDGE ( 'NONE', *, *, #18784, .T. ) ;
#9976=DIRECTION ( 'NONE',  ( 1.000000000000000000, 0.000000000000000000, 0.000000000000000000 ) ) ;
#9990=ORIENTED_EDGE ( 'NONE', *, *, #17001, .F. ) ;
#9991=VECTOR ( 'NONE', #11474, 1000.000000000000000 ) ;
#10065=ORIENTED_EDGE ( 'NONE', *, *, #11634, .T. ) ;
#10075=ORIENTED_EDGE ( 'NONE', *, *, #3400, .T. ) ;
#10079=FACE_OUTER_BOUND ( 'NONE', #15669, .T. ) ;
#10129=VECTOR ( 'NONE', #2703, 1000.000000000000000 ) ;
#10131=ORIENTED_EDGE ( 'NONE', *, *, #8453, .T. ) ;
#10133=LINE ( 'NONE', #20377, #21811 ) ;
#10151=AXIS2_PLACEMENT_3D ( 'NONE', #11625, #21450, #16255 ) ;
#10156=CYLINDRICAL_SURFACE ( 'NONE', #5634, 5.000000000000004441 ) ;
#10169=EDGE_CURVE ( 'NONE', #9454, #6320, #17030, .T. ) ;
#10177=ORIENTED_EDGE ( 'NONE', *, *, #11634, .F. ) ;
#10224=DIRECTION ( 'NONE',  ( 0.9385982292947090411, 0.3450121214752271959, -1.756657601269562932E-16 ) ) ;
#10237=EDGE_CURVE ( 'NONE', #10863, #15960, #16110, .T. ) ;
#10287=VECTOR ( 'NONE', #13787, 1000.000000000000000 ) ;
#10294=CIRCLE ( 'NONE', #20143, 5.000000000000004441 ) ;
#10302=STYLED_ITEM ( 'NONE', ( #16207 ), #14581 ) ;
#10307=CARTESIAN_POINT ( 'NONE',  ( 54.85617982533816672, 239.2521282348021714, -3.999999999999980904 ) ) ;
#10318=DIRECTION ( 'NONE',  ( 1.915514545828640458E-16, 7.041092946335503408E-17, 1.000000000000000000 ) ) ;
#10322=LINE ( 'NONE', #13721, #932 ) ;
#10323=ORIENTED_EDGE ( 'NONE', *, *, #988, .T. ) ;
#10329=LINE ( 'NONE', #5356, #6039 ) ;
#10348=ADVANCED_FACE ( 'NONE', ( #20677 ), #12616, .F. ) ;
#10360=CARTESIAN_POINT ( 'NONE',  ( -136.6255475934131596, 760.1741454933652449, -19.99999999999996092 ) ) ;
#10385=CARTESIAN_POINT ( 'NONE',  ( 111.4021762516569964, 137.5714195593754710, 4.000000000000003553 ) ) ;
#10393=VERTEX_POINT ( 'NONE', #15703 ) ;
#10415=CARTESIAN_POINT ( 'NONE',  ( -59.65946286876558702, 788.4655180356369328, -6.999999999999995559 ) ) ;
#10433=CARTESIAN_POINT ( 'NONE',  ( 147.5268905834513475, 193.0332408774651185, 272.0939500981630204 ) ) ;
#10438=VECTOR ( 'NONE', #19524, 1000.000000000000000 ) ;
#10442=DIRECTION ( 'NONE',  ( 0.9385982292947087080, 0.3450121214752276955, 0.000000000000000000 ) ) ;
#10490=VECTOR ( 'NONE', #7144, 1000.000000000000000 ) ;
#10499=CARTESIAN_POINT ( 'NONE',  ( 111.4021762516569964, 137.5714195593754710, -19.99999999999997868 ) ) ;
#10541=VECTOR ( 'NONE', #21461, 1000.000000000000000 ) ;
#10563=VERTEX_POINT ( 'NONE', #16455 ) ;
#10615=ORIENTED_EDGE ( 'NONE', *, *, #7850, .F. ) ;
#10633=VERTEX_POINT ( 'NONE', #11616 ) ;
#10644=CARTESIAN_POINT ( 'NONE',  ( -133.8097529055291943, 761.2091818577913500, -6.999999999999982236 ) ) ;
#10645=ORIENTED_EDGE ( 'NONE', *, *, #21469, .T. ) ;
#10648=CIRCLE ( 'NONE', #13460, 16.96660865288809816 ) ;
#10650=DIRECTION ( 'NONE',  ( -0.000000000000000000, -0.000000000000000000, -1.000000000000000000 ) ) ;
#10656=DIRECTION ( 'NONE',  ( 0.4874675571821264763, 0.8731411001063288380, -0.000000000000000000 ) ) ;
#10693=ORIENTED_EDGE ( 'NONE', *, *, #4382, .F. ) ;
#10694=EDGE_CURVE ( 'NONE', #19966, #2116, #17834, .T. ) ;
#10695=DIRECTION ( 'NONE',  ( 0.9385982292947089300, 0.3450121214752274734, 0.000000000000000000 ) ) ;
#10696=ORIENTED_EDGE ( 'NONE', *, *, #5177, .F. ) ;
#10722=ADVANCED_FACE ( 'NONE', ( #9540 ), #1257, .F. ) ;
#10744=CARTESIAN_POINT ( 'NONE',  ( 134.6380592378699532, 268.5785371414991687, -19.99999999999997868 ) ) ;
#10770=CARTESIAN_POINT ( 'NONE',  ( -56.84366818088135176, 789.5005544000622422, -19.99999999999997868 ) ) ;
#10803=EDGE_CURVE ( 'NONE', #21295, #5138, #19605, .T. ) ;
#10816=CARTESIAN_POINT ( 'NONE',  ( -56.84366818088135176, 789.5005544000622422, -19.99999999999997868 ) ) ;
#10823=EDGE_LOOP ( 'NONE', ( #18559, #19410, #10961, #21055 ) ) ;
#10830=ADVANCED_FACE ( 'NONE', ( #1999 ), #1590, .F. ) ;
#10837=AXIS2_PLACEMENT_3D ( 'NONE', #12350, #3986, #5841 ) ;
#10863=VERTEX_POINT ( 'NONE', #18969 ) ;
#10890=FACE_OUTER_BOUND ( 'NONE', #13427, .T. ) ;
#10910=ORIENTED_EDGE ( 'NONE', *, *, #6268, .F. ) ;
#10931=MECHANICAL_DESIGN_GEOMETRIC_PRESENTATION_REPRESENTATION('',(#15142),#16546);
#10961=ORIENTED_EDGE ( 'NONE', *, *, #15712, .F. ) ;
#10989=CARTESIAN_POINT ( 'NONE',  ( 96.62434152388762243, 220.7958015105191976, -5.999999999999976019 ) ) ;
#11008=EDGE_CURVE ( 'NONE', #1334, #10633, #13385, .T. ) ;
#11026=ORIENTED_EDGE ( 'NONE', *, *, #2682, .F. ) ;
#11054=DIRECTION ( 'NONE',  ( -0.9385982292947088190, -0.3450121214752274179, 0.000000000000000000 ) ) ;
#11057=ORIENTED_EDGE ( 'NONE', *, *, #10694, .F. ) ;
#11064=EDGE_CURVE ( 'NONE', #6320, #12307, #348, .T. ) ;
#11078=LINE ( 'NONE', #14273, #20911 ) ;
#11107=EDGE_CURVE ( 'NONE', #12991, #8122, #8701, .T. ) ;
#11134=ADVANCED_FACE ( 'NONE', ( #21384 ), #12455, .F. ) ;
#11141=ORIENTED_EDGE ( 'NONE', *, *, #5960, .T. ) ;
#11155=CARTESIAN_POINT ( 'NONE',  ( 54.85617982533816672, 239.2521282348021714, -3.999999999999980904 ) ) ;
#11221=CARTESIAN_POINT ( 'NONE',  ( 57.67197451322198276, 240.2871645992281628, -6.999999999999982236 ) ) ;
#11328=PRODUCT_DEFINITION_SHAPE ( 'NONE', 'NONE',  #15648 ) ;
#11333=EDGE_CURVE ( 'NONE', #1303, #16231, #16626, .T. ) ;
#11365=EDGE_CURVE ( 'NONE', #13557, #14220, #4839, .T. ) ;
#11367=CARTESIAN_POINT ( 'NONE',  ( 134.6380592378699532, 268.5785371414991687, -19.99999999999997868 ) ) ;
#11389=CARTESIAN_POINT ( 'NONE',  ( 147.5268905834513475, 193.0332408774651185, -19.99999999999997868 ) ) ;
#11445=FACE_OUTER_BOUND ( 'NONE', #7473, .T. ) ;
#11466=DIRECTION ( 'NONE',  ( -0.000000000000000000, 0.000000000000000000, -1.000000000000000000 ) ) ;
#11474=DIRECTION ( 'NONE',  ( 0.000000000000000000, 0.000000000000000000, 1.000000000000000000 ) ) ;
#11486=CIRCLE ( 'NONE', #15376, 10.00000000000000888 ) ;
#11497=DIRECTION ( 'NONE',  ( 0.3450121214752278065, -0.9385982292947087080, -0.000000000000000000 ) ) ;
#11550=FACE_OUTER_BOUND ( 'NONE', #15777, .T. ) ;
#11551=ORIENTED_EDGE ( 'NONE', *, *, #16699, .F. ) ;
#11594=DIRECTION ( 'NONE',  ( -0.9385982292947088190, -0.3450121214752274179, 2.040824802394967185E-16 ) ) ;
#11603=( GEOMETRIC_REPRESENTATION_CONTEXT ( 3 ) GLOBAL_UNCERTAINTY_ASSIGNED_CONTEXT ( ( #13497 ) ) GLOBAL_UNIT_ASSIGNED_CONTEXT ( ( #857, #4589, #12863 ) ) REPRESENTATION_CONTEXT ( 'NONE', 'WORKASPACE' ) );
#11612=CARTESIAN_POINT ( 'NONE',  ( 77.34521997529867576, 314.8592298662555322, 4.000000000000003553 ) ) ;
#11616=CARTESIAN_POINT ( 'NONE',  ( 139.9279279298906147, 262.8829071470229906, -5.999999999999976019 ) ) ;
#11625=CARTESIAN_POINT ( 'NONE',  ( 54.85617982533816672, 239.2521282348021714, -19.99999999999996092 ) ) ;
#11634=EDGE_CURVE ( 'NONE', #20857, #1303, #5255, .T. ) ;
#11665=CYLINDRICAL_SURFACE ( 'NONE', #11842, 10.00000000000000888 ) ;
#11680=CARTESIAN_POINT ( 'NONE',  ( 162.3411339277076308, 184.7625696037766261, -5.999999999999976019 ) ) ;
#11685=ORIENTED_EDGE ( 'NONE', *, *, #4149, .F. ) ;
#11698=DIRECTION ( 'NONE',  ( -0.8510798296367590998, -0.5250363069212118372, 0.000000000000000000 ) ) ;
#11710=LINE ( 'NONE', #18102, #3233 ) ;
#11726=DIRECTION ( 'NONE',  ( -0.000000000000000000, -0.000000000000000000, -1.000000000000000000 ) ) ;
#11742=EDGE_LOOP ( 'NONE', ( #14253, #15894, #11685, #2678 ) ) ;
#11748=CARTESIAN_POINT ( 'NONE',  ( 72.34521997529867576, 314.8592298662555322, 4.000000000000003553 ) ) ;
#11757=DIRECTION ( 'NONE',  ( 0.3450121214752274179, -0.9385982292947088190, 0.000000000000000000 ) ) ;
#11767=ORIENTED_EDGE ( 'NONE', *, *, #11107, .T. ) ;
#11798=ORIENTED_EDGE ( 'NONE', *, *, #13500, .F. ) ;
#11800=ORIENTED_EDGE ( 'NONE', *, *, #1784, .T. ) ;
#11829=ORIENTED_EDGE ( 'NONE', *, *, #17001, .T. ) ;
#11836=CARTESIAN_POINT ( 'NONE',  ( 54.85617982533818804, 239.2521282348021714, -19.99999999999996092 ) ) ;
#11842=AXIS2_PLACEMENT_3D ( 'NONE', #18403, #5066, #18289 ) ;
#11843=CIRCLE ( 'NONE', #7279, 10.00000000000000888 ) ;
#11851=CARTESIAN_POINT ( 'NONE',  ( 147.5268905834513475, 193.0332408774651185, -5.999999999999950262 ) ) ;
#11879=VERTEX_POINT ( 'NONE', #4902 ) ;
#11908=ORIENTED_EDGE ( 'NONE', *, *, #18980, .F. ) ;
#11925=ORIENTED_EDGE ( 'NONE', *, *, #3680, .T. ) ;
#11929=ORIENTED_EDGE ( 'NONE', *, *, #13773, .T. ) ;
#11934=ORIENTED_EDGE ( 'NONE', *, *, #4769, .F. ) ;
#11983=CYLINDRICAL_SURFACE ( 'NONE', #16012, 5.000000000000004441 ) ;
#12007=EDGE_LOOP ( 'NONE', ( #17641, #10177, #1894, #19468 ) ) ;
#12010=ADVANCED_FACE ( 'NONE', ( #16684 ), #7888, .T. ) ;
#12011=ORIENTED_EDGE ( 'NONE', *, *, #8895, .T. ) ;
#12025=LINE ( 'NONE', #8738, #10287 ) ;
#12035=VECTOR ( 'NONE', #6904, 1000.000000000000000 ) ;
#12088=FACE_OUTER_BOUND ( 'NONE', #9448, .T. ) ;
#12113=DIRECTION ( 'NONE',  ( -0.000000000000000000, -0.000000000000000000, -1.000000000000000000 ) ) ;
#12135=ORIENTED_EDGE ( 'NONE', *, *, #8887, .T. ) ;
#12161=CARTESIAN_POINT ( 'NONE',  ( 134.6380592378700101, 268.5785371414991687, -19.99999999999997868 ) ) ;
#12162=CARTESIAN_POINT ( 'NONE',  ( 130.1509106190733007, 127.1041540266590602, 272.0939500981630204 ) ) ;
#12164=ORIENTED_EDGE ( 'NONE', *, *, #17476, .F. ) ;
#12227=ORIENTED_EDGE ( 'NONE', *, *, #4382, .T. ) ;
#12242=DIRECTION ( 'NONE',  ( -1.000000000000000000, 0.000000000000000000, 0.000000000000000000 ) ) ;
#12260=CARTESIAN_POINT ( 'NONE',  ( 139.9279279298906147, 262.8829071470230474, 4.000000000000012434 ) ) ;
#12279=VERTEX_POINT ( 'NONE', #8437 ) ;
#12306=EDGE_CURVE ( 'NONE', #13533, #7143, #20657, .T. ) ;
#12307=VERTEX_POINT ( 'NONE', #15373 ) ;
#12350=CARTESIAN_POINT ( 'NONE',  ( 84.42064422693164261, 282.0082918409407284, -4.000000000000003553 ) ) ;
#12372=UNCERTAINTY_MEASURE_WITH_UNIT (LENGTH_MEASURE( 1.000000000000000082E-05 ), #8827, 'distance_accuracy_value', 'NONE');
#12378=VECTOR ( 'NONE', #9039, 1000.000000000000000 ) ;
#12396=AXIS2_PLACEMENT_3D ( 'NONE', #19385, #4495, #14633 ) ;
#12447=ORIENTED_EDGE ( 'NONE', *, *, #2945, .T. ) ;
#12455=PLANE ( 'NONE',  #17489 ) ;
#12507=CYLINDRICAL_SURFACE ( 'NONE', #4922, 10.00000000000000888 ) ;
#12555=DIRECTION ( 'NONE',  ( -0.3450121214752274179, 0.9385982292947088190, 0.000000000000000000 ) ) ;
#12558=AXIS2_PLACEMENT_3D ( 'NONE', #11389, #452, #9976 ) ;
#12564=DIRECTION ( 'NONE',  ( 1.000000000000000000, 0.000000000000000000, 0.000000000000000000 ) ) ;
#12567=DIRECTION ( 'NONE',  ( 1.000000000000000000, 0.000000000000000000, 0.000000000000000000 ) ) ;
#12574=EDGE_LOOP ( 'NONE', ( #5299, #18215 ) ) ;
#12607=LINE ( 'NONE', #10744, #276 ) ;
#12608=DIRECTION ( 'NONE',  ( 0.3450121214752278065, -0.9385982292947087080, -0.000000000000000000 ) ) ;
#12616=PLANE ( 'NONE',  #6634 ) ;
#12655=DIRECTION ( 'NONE',  ( 1.000000000000000000, 0.000000000000000000, 0.000000000000000000 ) ) ;
#12657=AXIS2_PLACEMENT_3D ( 'NONE', #2403, #7050, #17169 ) ;
#12667=CARTESIAN_POINT ( 'NONE',  ( 54.85617982533818804, 239.2521282348021714, -3.999999999999980904 ) ) ;
#12668=PRODUCT_DEFINITION_FORMATION_WITH_SPECIFIED_SOURCE ( 'ANY', '', #6419, .NOT_KNOWN. ) ;
#12749=AXIS2_PLACEMENT_3D ( 'NONE', #13736, #20474, #3718 ) ;
#12755=LINE ( 'NONE', #7483, #2641 ) ;
#12773=PLANE ( 'NONE',  #9835 ) ;
#12791=ORIENTED_EDGE ( 'NONE', *, *, #11107, .F. ) ;
#12803=CARTESIAN_POINT ( 'NONE',  ( 54.85617982533816672, 239.2521282348021714, -19.99999999999996092 ) ) ;
#12811=LINE ( 'NONE', #11155, #18914 ) ;
#12818=EDGE_LOOP ( 'NONE', ( #9631, #7444 ) ) ;
#12846=CARTESIAN_POINT ( 'NONE',  ( 163.4517194221884040, 198.8869265230379995, 272.0939500981630204 ) ) ;
#12854=ADVANCED_FACE ( 'NONE', ( #11550 ), #18279, .F. ) ;
#12863=( NAMED_UNIT ( * ) SI_UNIT ( $, .STERADIAN. ) SOLID_ANGLE_UNIT ( ) );
#12925=ORIENTED_EDGE ( 'NONE', *, *, #17954, .T. ) ;
#12932=DIRECTION ( 'NONE',  ( 0.000000000000000000, 0.000000000000000000, 1.000000000000000000 ) ) ;
#12940=AXIS2_PLACEMENT_3D ( 'NONE', #3180, #21704, #9909 ) ;
#12958=ORIENTED_EDGE ( 'NONE', *, *, #2399, .F. ) ;
#12985=LINE ( 'NONE', #6140, #14703 ) ;
#12991=VERTEX_POINT ( 'NONE', #11612 ) ;
#12996=FACE_OUTER_BOUND ( 'NONE', #15928, .T. ) ;
#13003=DIRECTION ( 'NONE',  ( -0.000000000000000000, -0.000000000000000000, -1.000000000000000000 ) ) ;
#13085=EDGE_CURVE ( 'NONE', #2592, #20857, #7882, .T. ) ;
#13104=AXIS2_PLACEMENT_3D ( 'NONE', #19174, #10695, #12555 ) ;
#13133=FACE_OUTER_BOUND ( 'NONE', #16787, .T. ) ;
#13155=EDGE_CURVE ( 'NONE', #4775, #7018, #16561, .T. ) ;
#13163=CARTESIAN_POINT ( 'NONE',  ( -59.65946286876558702, 788.4655180356369328, -19.99999999999997868 ) ) ;
#13220=CARTESIAN_POINT ( 'NONE',  ( 121.4021762516569964, 137.5714195593754710, 4.000000000000003553 ) ) ;
#13236=ORIENTED_EDGE ( 'NONE', *, *, #4149, .T. ) ;
#13242=CARTESIAN_POINT ( 'NONE',  ( -133.8097529055290522, 761.2091818577910090, -19.99999999999996092 ) ) ;
#13249=CARTESIAN_POINT ( 'NONE',  ( 134.6380592378699532, 268.5785371414991687, -3.999999999999996447 ) ) ;
#13266=ADVANCED_FACE ( 'NONE', ( #10079 ), #8644, .F. ) ;
#13321=ORIENTED_EDGE ( 'NONE', *, *, #13500, .T. ) ;
#13334=CYLINDRICAL_SURFACE ( 'NONE', #8672, 10.00000000000000888 ) ;
#13354=CIRCLE ( 'NONE', #1745, 5.000000000000004441 ) ;
#13385=LINE ( 'NONE', #15447, #15392 ) ;
#13398=VERTEX_POINT ( 'NONE', #20328 ) ;
#13399=DIRECTION ( 'NONE',  ( -0.000000000000000000, -0.000000000000000000, -1.000000000000000000 ) ) ;
#13403=CLOSED_SHELL ( 'NONE', ( #4668, #16986, #9320, #10830, #2995, #3355, #1069, #5684, #14740, #20166 ) ) ;
#13409=EDGE_CURVE ( 'NONE', #11879, #12307, #18562, .T. ) ;
#13419=DIRECTION ( 'NONE',  ( -0.9385982292947089300, -0.3450121214752274734, 0.000000000000000000 ) ) ;
#13427=EDGE_LOOP ( 'NONE', ( #10696, #1357, #169, #21754, #18636, #16661, #19801, #19490 ) ) ;
#13440=VECTOR ( 'NONE', #16437, 1000.000000000000000 ) ;
#13441=VECTOR ( 'NONE', #17449, 1000.000000000000000 ) ;
#13460=AXIS2_PLACEMENT_3D ( 'NONE', #13764, #17178, #3749 ) ;
#13482=DIRECTION ( 'NONE',  ( 0.3450121214752278065, -0.9385982292947087080, 0.000000000000000000 ) ) ;
#13485=VERTEX_POINT ( 'NONE', #15569 ) ;
#13494=DIRECTION ( 'NONE',  ( -0.3450121214752278620, 0.9385982292947087080, 0.000000000000000000 ) ) ;
#13497=UNCERTAINTY_MEASURE_WITH_UNIT (LENGTH_MEASURE( 1.000000000000000082E-05 ), #857, 'distance_accuracy_value', 'NONE');
#13500=EDGE_CURVE ( 'NONE', #5138, #21295, #11843, .T. ) ;
#13533=VERTEX_POINT ( 'NONE', #12260 ) ;
#13557=VERTEX_POINT ( 'NONE', #19205 ) ;
#13558=ORIENTED_EDGE ( 'NONE', *, *, #18980, .T. ) ;
#13609=FACE_OUTER_BOUND ( 'NONE', #17446, .T. ) ;
#13644=EDGE_CURVE ( 'NONE', #20857, #18306, #8966, .T. ) ;
#13664=PRESENTATION_STYLE_ASSIGNMENT (( #5292 ) ) ;
#13677=ADVANCED_FACE ( 'NONE', ( #13133, #4313, #14450 ), #19637, .T. ) ;
#13708=CARTESIAN_POINT ( 'NONE',  ( 89.42064422693164261, 282.0082918409407284, -4.000000000000004441 ) ) ;
#13721=CARTESIAN_POINT ( 'NONE',  ( 54.85617982533818804, 239.2521282348021714, -3.999999999999980904 ) ) ;
#13730=PLANE ( 'NONE',  #5801 ) ;
#13736=CARTESIAN_POINT ( 'NONE',  ( 147.5268905834513475, 193.0332408774651185, 272.0939500981630204 ) ) ;
#13738=EDGE_CURVE ( 'NONE', #255, #2224, #17970, .T. ) ;
#13764=CARTESIAN_POINT ( 'NONE',  ( 147.5268905834513475, 193.0332408774651185, -19.99999999999997868 ) ) ;
#13773=EDGE_CURVE ( 'NONE', #5574, #2417, #4416, .T. ) ;
#13787=DIRECTION ( 'NONE',  ( 0.000000000000000000, 0.000000000000000000, 1.000000000000000000 ) ) ;
#13865=CARTESIAN_POINT ( 'NONE',  ( 121.4021762516569964, 137.5714195593754710, -19.99999999999997868 ) ) ;
#13889=CARTESIAN_POINT ( 'NONE',  ( 101.4021762516569822, 137.5714195593754710, 4.000000000000003553 ) ) ;
#13908=DIRECTION ( 'NONE',  ( 0.000000000000000000, 0.000000000000000000, 1.000000000000000000 ) ) ;
#13927=ORIENTED_EDGE ( 'NONE', *, *, #13155, .F. ) ;
#13957=DIRECTION ( 'NONE',  ( -0.3450121214752274734, 0.9385982292947089300, 0.000000000000000000 ) ) ;
#13962=DIRECTION ( 'NONE',  ( 0.000000000000000000, 0.000000000000000000, 1.000000000000000000 ) ) ;
#13979=CARTESIAN_POINT ( 'NONE',  ( 111.4021762516569964, 137.5714195593754710, -19.99999999999997868 ) ) ;
#14019=DIRECTION ( 'NONE',  ( 1.000000000000000000, 0.000000000000000000, 0.000000000000000000 ) ) ;
#14046=EDGE_CURVE ( 'NONE', #7555, #17533, #8667, .T. ) ;
#14148=ORIENTED_EDGE ( 'NONE', *, *, #12306, .T. ) ;
#14159=EDGE_CURVE ( 'NONE', #20087, #1303, #10322, .T. ) ;
#14169=CARTESIAN_POINT ( 'NONE',  ( 101.6431471920911207, 239.2647937927896464, -5.999999999999976019 ) ) ;
#14171=CARTESIAN_POINT ( 'NONE',  ( 77.34521997529867576, 314.8592298662555322, -4.000000000000004441 ) ) ;
#14185=DIRECTION ( 'NONE',  ( 0.9385982292947090411, 0.3450121214752271959, -1.756657601269562932E-16 ) ) ;
#14214=DIRECTION ( 'NONE',  ( 1.000000000000000000, 0.000000000000000000, 0.000000000000000000 ) ) ;
#14220=VERTEX_POINT ( 'NONE', #10644 ) ;
#14229=ORIENTED_EDGE ( 'NONE', *, *, #11333, .F. ) ;
#14242=ORIENTED_EDGE ( 'NONE', *, *, #2399, .T. ) ;
#14253=ORIENTED_EDGE ( 'NONE', *, *, #5368, .T. ) ;
#14273=CARTESIAN_POINT ( 'NONE',  ( 67.34521997529867576, 314.8592298662555322, 272.0939500981630204 ) ) ;
#14298=CIRCLE ( 'NONE', #20314, 5.000000000000004441 ) ;
#14304=VECTOR ( 'NONE', #11497, 1000.000000000000114 ) ;
#14331=ORIENTED_EDGE ( 'NONE', *, *, #1239, .F. ) ;
#14343=VECTOR ( 'NONE', #13399, 1000.000000000000000 ) ;
#14347=VECTOR ( 'NONE', #2030, 1000.000000000000114 ) ;
#14373=CARTESIAN_POINT ( 'NONE',  ( 93.25569916848381524, 126.0916958004080755, 4.000000000000003553 ) ) ;
#14450=FACE_BOUND ( 'NONE', #21019, .T. ) ;
#14470=ORIENTED_EDGE ( 'NONE', *, *, #9771, .T. ) ;
#14487=EDGE_CURVE ( 'NONE', #9553, #9751, #14578, .T. ) ;
#14499=MECHANICAL_DESIGN_GEOMETRIC_PRESENTATION_REPRESENTATION('',(#10302),#4656);
#14530=DIRECTION ( 'NONE',  ( -0.000000000000000000, -0.000000000000000000, -1.000000000000000000 ) ) ;
#14543=FACE_OUTER_BOUND ( 'NONE', #10823, .T. ) ;
#14557=DIRECTION ( 'NONE',  ( 0.000000000000000000, 0.000000000000000000, 1.000000000000000000 ) ) ;
#14578=LINE ( 'NONE', #2794, #20660 ) ;
#14581=MANIFOLD_SOLID_BREP ( 'Cut-Extrude9', #20437 ) ;
#14590=DIRECTION ( 'NONE',  ( -0.000000000000000000, -0.000000000000000000, -1.000000000000000000 ) ) ;
#14633=DIRECTION ( 'NONE',  ( 1.000000000000000000, 0.000000000000000000, -1.734723475976805615E-16 ) ) ;
#14648=AXIS2_PLACEMENT_3D ( 'NONE', #6782, #7100, #21767 ) ;
#14703=VECTOR ( 'NONE', #6254, 1000.000000000000114 ) ;
#14704=CARTESIAN_POINT ( 'NONE',  ( 111.4021762516569964, 137.5714195593754710, 272.0939500981630204 ) ) ;
#14714=FACE_OUTER_BOUND ( 'NONE', #7463, .T. ) ;
#14740=ADVANCED_FACE ( 'NONE', ( #18847 ), #8721, .F. ) ;
#14742=DIRECTION ( 'NONE',  ( -0.3450121214752274179, 0.9385982292947088190, -0.000000000000000000 ) ) ;
#14827=DIRECTION ( 'NONE',  ( -0.000000000000000000, -0.000000000000000000, 1.000000000000000000 ) ) ;
#14877=FACE_OUTER_BOUND ( 'NONE', #5875, .T. ) ;
#14906=ORIENTED_EDGE ( 'NONE', *, *, #11365, .T. ) ;
#14915=LINE ( 'NONE', #3358, #429 ) ;
#14959=EDGE_LOOP ( 'NONE', ( #8858, #11057 ) ) ;
#14969=FACE_OUTER_BOUND ( 'NONE', #12007, .T. ) ;
#15000=EDGE_CURVE ( 'NONE', #4862, #13398, #3954, .T. ) ;
#15002=CARTESIAN_POINT ( 'NONE',  ( 109.8528842077358405, 344.7014318495014322, 272.0939500981630204 ) ) ;
#15011=VECTOR ( 'NONE', #6838, 1000.000000000000000 ) ;
#15042=VECTOR ( 'NONE', #8193, 1000.000000000000000 ) ;
#15043=PLANE ( 'NONE',  #10151 ) ;
#15081=DIRECTION ( 'NONE',  ( 1.723963091245776585E-16, 6.336983651701954299E-17, 1.000000000000000000 ) ) ;
#15102=DIRECTION ( 'NONE',  ( -1.000000000000000000, 0.000000000000000000, 0.000000000000000000 ) ) ;
#15109=VECTOR ( 'NONE', #19955, 1000.000000000000114 ) ;
#15120=LINE ( 'NONE', #3659, #19618 ) ;
#15142=STYLED_ITEM ( 'NONE', ( #13664 ), #283 ) ;
#15154=EDGE_CURVE ( 'NONE', #7040, #21732, #16905, .T. ) ;
#15256=CARTESIAN_POINT ( 'NONE',  ( -59.65946286876558702, 788.4655180356369328, -6.999999999999995559 ) ) ;
#15298=DIRECTION ( 'NONE',  ( -1.000000000000000000, 0.000000000000000000, 0.000000000000000000 ) ) ;
#15371=LINE ( 'NONE', #264, #15561 ) ;
#15373=CARTESIAN_POINT ( 'NONE',  ( 24.43941541943582862, 313.3049502139530205, -19.99999999999997868 ) ) ;
#15376=AXIS2_PLACEMENT_3D ( 'NONE', #13979, #538, #758 ) ;
#15377=AXIS2_PLACEMENT_3D ( 'NONE', #1451, #11466, #19860 ) ;
#15392=VECTOR ( 'NONE', #7298, 1000.000000000000114 ) ;
#15395=DIRECTION ( 'NONE',  ( 0.000000000000000000, 0.000000000000000000, 1.000000000000000000 ) ) ;
#15447=CARTESIAN_POINT ( 'NONE',  ( 163.4517194221884040, 198.8869265230379995, -5.999999999999976019 ) ) ;
#15449=EDGE_CURVE ( 'NONE', #12991, #8176, #21199, .T. ) ;
#15478=FACE_OUTER_BOUND ( 'NONE', #1634, .T. ) ;
#15498=DIRECTION ( 'NONE',  ( -0.9385982292947087080, -0.3450121214752276955, -0.000000000000000000 ) ) ;
#15513=CARTESIAN_POINT ( 'NONE',  ( -70.94676665037202667, 193.0091883945747213, 0.000000000000000000 ) ) ;
#15535=( NAMED_UNIT ( * ) PLANE_ANGLE_UNIT ( ) SI_UNIT ( $, .RADIAN. ) );
#15537=ORIENTED_EDGE ( 'NONE', *, *, #9429, .T. ) ;
#15561=VECTOR ( 'NONE', #18675, 999.9999999999998863 ) ;
#15565=ORIENTED_EDGE ( 'NONE', *, *, #14046, .F. ) ;
#15568=DIRECTION ( 'NONE',  ( 1.000000000000000000, 0.000000000000000000, -0.000000000000000000 ) ) ;
#15569=CARTESIAN_POINT ( 'NONE',  ( 93.25569916848381524, 126.0916958004080755, 4.000000000000003553 ) ) ;
#15612=DIRECTION ( 'NONE',  ( -0.9385982292947088190, -0.3450121214752274179, 0.000000000000000000 ) ) ;
#15639=ORIENTED_EDGE ( 'NONE', *, *, #14046, .T. ) ;
#15648=PRODUCT_DEFINITION ( 'UNKNOWN', '', #12668, #6655 ) ;
#15661=VERTEX_POINT ( 'NONE', #16985 ) ;
#15664=ADVANCED_FACE ( 'NONE', ( #5314 ), #16771, .F. ) ;
#15669=EDGE_LOOP ( 'NONE', ( #4913, #20590, #11829, #21101 ) ) ;
#15671=CARTESIAN_POINT ( 'NONE',  ( 108.9927164799167372, 227.3511983043831037, 4.000000000000021316 ) ) ;
#15672=CARTESIAN_POINT ( 'NONE',  ( -56.84366818088135176, 789.5005544000622422, -3.999999999999996447 ) ) ;
#15703=CARTESIAN_POINT ( 'NONE',  ( 130.1509106190733007, 127.1041540266590602, -19.99999999999997868 ) ) ;
#15712=EDGE_CURVE ( 'NONE', #2417, #13557, #12025, .T. ) ;
#15724=AXIS2_PLACEMENT_3D ( 'NONE', #8673, #15395, #720 ) ;
#15763=DIRECTION ( 'NONE',  ( 0.000000000000000000, 0.000000000000000000, 1.000000000000000000 ) ) ;
#15777=EDGE_LOOP ( 'NONE', ( #9662, #9773, #21288, #2600 ) ) ;
#15894=ORIENTED_EDGE ( 'NONE', *, *, #16496, .T. ) ;
#15928=EDGE_LOOP ( 'NONE', ( #21542, #1503, #14331, #14906 ) ) ;
#15930=EDGE_CURVE ( 'NONE', #9805, #9751, #2172, .T. ) ;
#15960=VERTEX_POINT ( 'NONE', #20848 ) ;
#15973=DIRECTION ( 'NONE',  ( 1.000000000000000000, 0.000000000000000000, -1.915514545828640458E-16 ) ) ;
#15986=ORIENTED_EDGE ( 'NONE', *, *, #15154, .F. ) ;
#16012=AXIS2_PLACEMENT_3D ( 'NONE', #6601, #17154, #15298 ) ;
#16040=ORIENTED_EDGE ( 'NONE', *, *, #16699, .T. ) ;
#16071=DIRECTION ( 'NONE',  ( 1.000000000000000000, 0.000000000000000000, 0.000000000000000000 ) ) ;
#16087=AXIS2_PLACEMENT_3D ( 'NONE', #11851, #3486, #1826 ) ;
#16101=ORIENTED_EDGE ( 'NONE', *, *, #1239, .T. ) ;
#16110=CIRCLE ( 'NONE', #15724, 13.99821153497579651 ) ;
#16125=LINE ( 'NONE', #16228, #7621 ) ;
#16149=LINE ( 'NONE', #17795, #10129 ) ;
#16170=CARTESIAN_POINT ( 'NONE',  ( 147.5268905834513475, 193.0332408774651185, -5.999999999999950262 ) ) ;
#16187=DIRECTION ( 'NONE',  ( 0.000000000000000000, 0.000000000000000000, 1.000000000000000000 ) ) ;
#16204=ORIENTED_EDGE ( 'NONE', *, *, #3400, .F. ) ;
#16207=PRESENTATION_STYLE_ASSIGNMENT (( #9510 ) ) ;
#16228=CARTESIAN_POINT ( 'NONE',  ( 93.25569916848381524, 126.0916958004080755, 272.0939500981630204 ) ) ;
#16229=CARTESIAN_POINT ( 'NONE',  ( -56.84366818088135176, 789.5005544000622422, -19.99999999999997868 ) ) ;
#16231=VERTEX_POINT ( 'NONE', #12161 ) ;
#16236=DIRECTION ( 'NONE',  ( 0.9385982292947088190, 0.3450121214752274179, -1.836742322155470491E-16 ) ) ;
#16241=CARTESIAN_POINT ( 'NONE',  ( 72.34521997529867576, 314.8592298662555322, 272.0939500981630204 ) ) ;
#16255=DIRECTION ( 'NONE',  ( 0.3450121214752278065, -0.9385982292947087080, 0.000000000000000000 ) ) ;
#16267=LINE ( 'NONE', #10989, #8444 ) ;
#16276=CARTESIAN_POINT ( 'NONE',  ( 134.6380592378699532, 268.5785371414991687, -3.999999999999996447 ) ) ;
#16306=ORIENTED_EDGE ( 'NONE', *, *, #9461, .T. ) ;
#16369=ORIENTED_EDGE ( 'NONE', *, *, #5960, .F. ) ;
#16384=CARTESIAN_POINT ( 'NONE',  ( 89.42064422693164261, 282.0082918409407284, 272.0939500981630204 ) ) ;
#16396=CARTESIAN_POINT ( 'NONE',  ( 101.4021762516569822, 137.5714195593754710, 272.0939500981630204 ) ) ;
#16404=CARTESIAN_POINT ( 'NONE',  ( 57.67197451322198276, 240.2871645992281628, -6.999999999999982236 ) ) ;
#16407=VECTOR ( 'NONE', #13003, 1000.000000000000000 ) ;
#16423=ORIENTED_EDGE ( 'NONE', *, *, #13738, .T. ) ;
#16437=DIRECTION ( 'NONE',  ( -0.000000000000000000, -0.000000000000000000, -1.000000000000000000 ) ) ;
#16455=CARTESIAN_POINT ( 'NONE',  ( 107.0370895198517189, 343.6663954850758955, -19.99999999999997868 ) ) ;
#16479=EDGE_CURVE ( 'NONE', #5574, #14220, #2251, .T. ) ;
#16484=FACE_OUTER_BOUND ( 'NONE', #16890, .T. ) ;
#16496=EDGE_CURVE ( 'NONE', #17982, #21732, #20773, .T. ) ;
#16546=( GEOMETRIC_REPRESENTATION_CONTEXT ( 3 ) GLOBAL_UNCERTAINTY_ASSIGNED_CONTEXT ( ( #12372 ) ) GLOBAL_UNIT_ASSIGNED_CONTEXT ( ( #8827, #15535, #7062 ) ) REPRESENTATION_CONTEXT ( 'NONE', 'WORKASPACE' ) );
#16561=LINE ( 'NONE', #2797, #14304 ) ;
#16565=DIRECTION ( 'NONE',  ( -0.000000000000000000, -0.000000000000000000, -1.000000000000000000 ) ) ;
#16584=EDGE_LOOP ( 'NONE', ( #2650, #2221, #17742, #19223, #5057, #21764, #6085, #14242 ) ) ;
#16612=VECTOR ( 'NONE', #19619, 1000.000000000000000 ) ;
#16618=DIRECTION ( 'NONE',  ( 0.000000000000000000, 0.000000000000000000, -1.000000000000000000 ) ) ;
#16626=LINE ( 'NONE', #9704, #3774 ) ;
#16661=ORIENTED_EDGE ( 'NONE', *, *, #6688, .T. ) ;
#16669=DIRECTION ( 'NONE',  ( -0.9385982292947088190, -0.3450121214752278620, 0.000000000000000000 ) ) ;
#16684=FACE_OUTER_BOUND ( 'NONE', #18528, .T. ) ;
#16699=EDGE_CURVE ( 'NONE', #2116, #13398, #17878, .T. ) ;
#16771=PLANE ( 'NONE',  #9576 ) ;
#16774=EDGE_CURVE ( 'NONE', #18306, #16231, #2904, .T. ) ;
#16787=EDGE_LOOP ( 'NONE', ( #6401, #10910, #3003, #8226, #2547, #2976, #9990, #8883, #6743, #11934 ) ) ;
#16810=DIRECTION ( 'NONE',  ( -0.3450121214752278065, 0.9385982292947087080, -0.000000000000000000 ) ) ;
#16871=LINE ( 'NONE', #15002, #4773 ) ;
#16890=EDGE_LOOP ( 'NONE', ( #899, #20995, #7824, #11141 ) ) ;
#16905=LINE ( 'NONE', #10415, #9247 ) ;
#16914=EDGE_CURVE ( 'NONE', #15661, #2045, #11710, .T. ) ;
#16919=EDGE_LOOP ( 'NONE', ( #7234, #12925, #17289, #10693 ) ) ;
#16924=DIRECTION ( 'NONE',  ( 0.000000000000000000, 0.000000000000000000, 1.000000000000000000 ) ) ;
#16985=CARTESIAN_POINT ( 'NONE',  ( 130.1509106190733007, 127.1041540266590602, 4.000000000000003553 ) ) ;
#16986=ADVANCED_FACE ( 'NONE', ( #18217 ), #3011, .F. ) ;
#17001=EDGE_CURVE ( 'NONE', #12307, #120, #20000, .T. ) ;
#17010=CYLINDRICAL_SURFACE ( 'NONE', #19222, 5.000000000000004441 ) ;
#17020=DIRECTION ( 'NONE',  ( 1.000000000000000000, 0.000000000000000000, -1.915514545828640458E-16 ) ) ;
#17024=DIRECTION ( 'NONE',  ( 0.9385982292947088190, 0.3450121214752274179, -1.836742322155470491E-16 ) ) ;
#17030=LINE ( 'NONE', #1838, #7291 ) ;
#17077=VERTEX_POINT ( 'NONE', #18333 ) ;
#17104=VECTOR ( 'NONE', #14557, 1000.000000000000000 ) ;
#17139=AXIS2_PLACEMENT_3D ( 'NONE', #3590, #10318, #17020 ) ;
#17142=LINE ( 'NONE', #6814, #6884 ) ;
#17154=DIRECTION ( 'NONE',  ( -0.000000000000000000, -0.000000000000000000, -1.000000000000000000 ) ) ;
#17169=DIRECTION ( 'NONE',  ( 1.000000000000000000, 0.000000000000000000, 0.000000000000000000 ) ) ;
#17170=FACE_BOUND ( 'NONE', #8830, .T. ) ;
#17178=DIRECTION ( 'NONE',  ( 0.000000000000000000, 0.000000000000000000, 1.000000000000000000 ) ) ;
#17219=UNCERTAINTY_MEASURE_WITH_UNIT (LENGTH_MEASURE( 1.000000000000000082E-05 ), #19634, 'distance_accuracy_value', 'NONE');
#17223=CIRCLE ( 'NONE', #18291, 16.96660865288809816 ) ;
#17284=CARTESIAN_POINT ( 'NONE',  ( 96.62434152388763664, 220.7958015105191976, -5.999999999999976019 ) ) ;
#17289=ORIENTED_EDGE ( 'NONE', *, *, #17669, .T. ) ;
#17424=ORIENTED_EDGE ( 'NONE', *, *, #7850, .T. ) ;
#17427=VERTEX_POINT ( 'NONE', #11680 ) ;
#17445=VECTOR ( 'NONE', #9951, 1000.000000000000000 ) ;
#17446=EDGE_LOOP ( 'NONE', ( #9183, #11929, #6075, #13927 ) ) ;
#17449=DIRECTION ( 'NONE',  ( 0.000000000000000000, 0.000000000000000000, 1.000000000000000000 ) ) ;
#17457=AXIS2_PLACEMENT_3D ( 'NONE', #6383, #4725, #18171 ) ;
#17468=SHAPE_REPRESENTATION ( 'Handle Grip', ( #12657 ), #11603 ) ;
#17476=EDGE_CURVE ( 'NONE', #2417, #7018, #20288, .T. ) ;
#17489=AXIS2_PLACEMENT_3D ( 'NONE', #9374, #2424, #19184 ) ;
#17502=VECTOR ( 'NONE', #6454, 1000.000000000000000 ) ;
#17533=VERTEX_POINT ( 'NONE', #9149 ) ;
#17549=EDGE_CURVE ( 'NONE', #15960, #17077, #2297, .T. ) ;
#17582=ORIENTED_EDGE ( 'NONE', *, *, #15449, .F. ) ;
#17600=COLOUR_RGB ( '', 0.31764706, 0.68627451, 0.89019608) ;
#17627=CARTESIAN_POINT ( 'NONE',  ( 111.4021762516569964, 137.5714195593754710, 4.000000000000003553 ) ) ;
#17637=ORIENTED_EDGE ( 'NONE', *, *, #17954, .F. ) ;
#17641=ORIENTED_EDGE ( 'NONE', *, *, #14159, .T. ) ;
#17642=VECTOR ( 'NONE', #9532, 1000.000000000000000 ) ;
#17669=EDGE_CURVE ( 'NONE', #12279, #1240, #10648, .T. ) ;
#17689=DIRECTION ( 'NONE',  ( -0.000000000000000000, -0.000000000000000000, -1.000000000000000000 ) ) ;
#17714=CARTESIAN_POINT ( 'NONE',  ( 131.8222645499855901, 267.5435007770738025, -6.999999999999995559 ) ) ;
#17720=VERTEX_POINT ( 'NONE', #2619 ) ;
#17722=CARTESIAN_POINT ( 'NONE',  ( 89.42064422693164261, 282.0082918409407284, 4.000000000000003553 ) ) ;
#17742=ORIENTED_EDGE ( 'NONE', *, *, #20930, .F. ) ;
#17795=CARTESIAN_POINT ( 'NONE',  ( 139.9279279298906147, 262.8829071470229906, -5.999999999999976019 ) ) ;
#17821=EDGE_CURVE ( 'NONE', #19772, #7040, #6255, .T. ) ;
#17834=CIRCLE ( 'NONE', #19263, 5.000000000000004441 ) ;
#17858=SURFACE_STYLE_FILL_AREA ( #4413 ) ;
#17869=LINE ( 'NONE', #4653, #15042 ) ;
#17878=LINE ( 'NONE', #9418, #17642 ) ;
#17910=ORIENTED_EDGE ( 'NONE', *, *, #16479, .F. ) ;
#17919=CARTESIAN_POINT ( 'NONE',  ( 108.9927164799167372, 227.3511983043831037, -5.999999999999976019 ) ) ;
#17951=FACE_OUTER_BOUND ( 'NONE', #11742, .T. ) ;
#17954=EDGE_CURVE ( 'NONE', #17427, #12279, #14915, .T. ) ;
#17970=LINE ( 'NONE', #12803, #17104 ) ;
#17982=VERTEX_POINT ( 'NONE', #156 ) ;
#18040=DIRECTION ( 'NONE',  ( -0.000000000000000000, -0.000000000000000000, -1.000000000000000000 ) ) ;
#18056=EDGE_CURVE ( 'NONE', #13533, #9454, #15371, .T. ) ;
#18086=VECTOR ( 'NONE', #2083, 1000.000000000000000 ) ;
#18102=CARTESIAN_POINT ( 'NONE',  ( 162.3411339277076308, 184.7625696037766261, 4.000000000000003553 ) ) ;
#18103=ADVANCED_FACE ( 'NONE', ( #8323 ), #20439, .T. ) ;
#18104=AXIS2_PLACEMENT_3D ( 'NONE', #15671, #3894, #16071 ) ;
#18132=ORIENTED_EDGE ( 'NONE', *, *, #4408, .T. ) ;
#18171=DIRECTION ( 'NONE',  ( -1.000000000000000000, 0.000000000000000000, 1.723963091245776092E-16 ) ) ;
#18192=ORIENTED_EDGE ( 'NONE', *, *, #3680, .F. ) ;
#18215=ORIENTED_EDGE ( 'NONE', *, *, #7644, .F. ) ;
#18216=CARTESIAN_POINT ( 'NONE',  ( 111.4021762516569964, 137.5714195593754710, 4.000000000000003553 ) ) ;
#18217=FACE_OUTER_BOUND ( 'NONE', #20374, .T. ) ;
#18224=EDGE_LOOP ( 'NONE', ( #2013, #5223, #21483, #18792 ) ) ;
#18233=CARTESIAN_POINT ( 'NONE',  ( -70.94676665037205510, 193.0091883945745792, 0.000000000000000000 ) ) ;
#18268=LINE ( 'NONE', #16384, #4780 ) ;
#18279=PLANE ( 'NONE',  #12940 ) ;
#18289=DIRECTION ( 'NONE',  ( -1.000000000000000000, 0.000000000000000000, 0.000000000000000000 ) ) ;
#18291=AXIS2_PLACEMENT_3D ( 'NONE', #1424, #1312, #8047 ) ;
#18306=VERTEX_POINT ( 'NONE', #3900 ) ;
#18320=LINE ( 'NONE', #18542, #474 ) ;
#18333=CARTESIAN_POINT ( 'NONE',  ( 138.4260920561042667, 141.9264758756783351, -5.999999999999976019 ) ) ;
#18403=CARTESIAN_POINT ( 'NONE',  ( 111.4021762516569964, 137.5714195593754710, 272.0939500981630204 ) ) ;
#18437=EDGE_CURVE ( 'NONE', #5574, #4775, #2779, .T. ) ;
#18460=PLANE ( 'NONE',  #6545 ) ;
#18508=CARTESIAN_POINT ( 'NONE',  ( 134.6380592378699532, 268.5785371414991687, -19.99999999999997868 ) ) ;
#18528=EDGE_LOOP ( 'NONE', ( #11026, #1778, #8287, #1025 ) ) ;
#18537=VECTOR ( 'NONE', #8318, 1000.000000000000227 ) ;
#18539=CARTESIAN_POINT ( 'NONE',  ( 57.67197451322198276, 240.2871645992281628, -19.99999999999997868 ) ) ;
#18542=CARTESIAN_POINT ( 'NONE',  ( 139.9279279298906147, 262.8829071470229906, -5.999999999999976019 ) ) ;
#18546=DIRECTION ( 'NONE',  ( -0.8731411001063289490, 0.4874675571821265319, 0.000000000000000000 ) ) ;
#18553=ORIENTED_EDGE ( 'NONE', *, *, #5368, .F. ) ;
#18559=ORIENTED_EDGE ( 'NONE', *, *, #16479, .T. ) ;
#18562=LINE ( 'NONE', #1587, #18537 ) ;
#18633=SURFACE_SIDE_STYLE ('',( #117 ) ) ;
#18636=ORIENTED_EDGE ( 'NONE', *, *, #10169, .T. ) ;
#18665=ORIENTED_EDGE ( 'NONE', *, *, #15930, .F. ) ;
#18675=DIRECTION ( 'NONE',  ( -0.3450121214752277510, 0.9385982292947088190, 0.000000000000000000 ) ) ;
#18755=DIRECTION ( 'NONE',  ( 1.000000000000000000, 0.000000000000000000, 0.000000000000000000 ) ) ;
#18773=ORIENTED_EDGE ( 'NONE', *, *, #17549, .T. ) ;
#18784=EDGE_CURVE ( 'NONE', #17077, #2045, #8945, .T. ) ;
#18792=ORIENTED_EDGE ( 'NONE', *, *, #16496, .F. ) ;
#18804=AXIS2_PLACEMENT_3D ( 'NONE', #17627, #20952, #12567 ) ;
#18807=DIRECTION ( 'NONE',  ( 0.3450121214752277510, -0.9385982292947088190, 0.000000000000000000 ) ) ;
#18847=FACE_OUTER_BOUND ( 'NONE', #18224, .T. ) ;
#18906=VECTOR ( 'NONE', #1315, 1000.000000000000227 ) ;
#18914=VECTOR ( 'NONE', #2891, 1000.000000000000114 ) ;
#18927=ORIENTED_EDGE ( 'NONE', *, *, #7316, .T. ) ;
#18936=ADVANCED_FACE ( 'NONE', ( #4618 ), #6274, .T. ) ;
#18948=CARTESIAN_POINT ( 'NONE',  ( 101.4021762516569822, 137.5714195593754710, -19.99999999999997868 ) ) ;
#18960=ORIENTED_EDGE ( 'NONE', *, *, #16914, .F. ) ;
#18969=CARTESIAN_POINT ( 'NONE',  ( 101.6431471920911207, 239.2647937927896464, -5.999999999999976019 ) ) ;
#18971=DIRECTION ( 'NONE',  ( -0.000000000000000000, -0.000000000000000000, 1.000000000000000000 ) ) ;
#18980=EDGE_CURVE ( 'NONE', #2626, #9553, #165, .T. ) ;
#18993=PLANE ( 'NONE',  #5945 ) ;
#19012=CARTESIAN_POINT ( 'NONE',  ( -59.65946286876545201, 788.4655180356365918, -19.99999999999997868 ) ) ;
#19026=DIRECTION ( 'NONE',  ( 0.3450121214752278065, -0.9385982292947087080, -0.000000000000000000 ) ) ;
#19046=DIRECTION ( 'NONE',  ( 1.000000000000000000, 0.000000000000000000, -0.000000000000000000 ) ) ;
#19055=CARTESIAN_POINT ( 'NONE',  ( 137.5268905834513191, 193.0332408774651185, -5.999999999999950262 ) ) ;
#19073=VECTOR ( 'NONE', #12608, 1000.000000000000114 ) ;
#19146=PLANE ( 'NONE',  #21675 ) ;
#19158=FACE_BOUND ( 'NONE', #12818, .T. ) ;
#19173=EDGE_CURVE ( 'NONE', #9746, #21295, #20073, .T. ) ;
#19174=CARTESIAN_POINT ( 'NONE',  ( 131.8222645499855901, 267.5435007770738025, -6.999999999999995559 ) ) ;
#19184=DIRECTION ( 'NONE',  ( -0.3450121214752278065, 0.9385982292947087080, 0.000000000000000000 ) ) ;
#19191=CARTESIAN_POINT ( 'NONE',  ( -133.8097529055291943, 761.2091818577913500, -19.99999999999997868 ) ) ;
#19205=CARTESIAN_POINT ( 'NONE',  ( 57.67197451322198276, 240.2871645992281628, -6.999999999999982236 ) ) ;
#19222=AXIS2_PLACEMENT_3D ( 'NONE', #1917, #11726, #19399 ) ;
#19223=ORIENTED_EDGE ( 'NONE', *, *, #3835, .F. ) ;
#19233=DIRECTION ( 'NONE',  ( -1.000000000000000000, 0.000000000000000000, 0.000000000000000000 ) ) ;
#19246=DIRECTION ( 'NONE',  ( -0.000000000000000000, -0.000000000000000000, 1.000000000000000000 ) ) ;
#19263=AXIS2_PLACEMENT_3D ( 'NONE', #2686, #9431, #4561 ) ;
#19300=DIRECTION ( 'NONE',  ( 0.000000000000000000, 0.000000000000000000, 1.000000000000000000 ) ) ;
#19305=ADVANCED_FACE ( 'NONE', ( #17170, #19158, #21254 ), #1077, .F. ) ;
#19317=DIRECTION ( 'NONE',  ( -0.9385982292947088190, -0.3450121214752274179, 2.040824802394967185E-16 ) ) ;
#19328=DIRECTION ( 'NONE',  ( -0.9385982292947087080, -0.3450121214752278620, 2.040824802394967678E-16 ) ) ;
#19363=CARTESIAN_POINT ( 'NONE',  ( 131.4397495910615135, 111.2323268066561894, 4.000000000000021316 ) ) ;
#19385=CARTESIAN_POINT ( 'NONE',  ( 84.42064422693164261, 282.0082918409407284, -4.000000000000003553 ) ) ;
#19396=DIRECTION ( 'NONE',  ( -1.000000000000000000, 0.000000000000000000, 0.000000000000000000 ) ) ;
#19399=DIRECTION ( 'NONE',  ( -1.000000000000000000, 0.000000000000000000, 0.000000000000000000 ) ) ;
#19410=ORIENTED_EDGE ( 'NONE', *, *, #11365, .F. ) ;
#19428=VECTOR ( 'NONE', #14742, 1000.000000000000227 ) ;
#19436=CARTESIAN_POINT ( 'NONE',  ( -262.4284940691233601, 713.9312056531377948, 0.000000000000000000 ) ) ;
#19460=CARTESIAN_POINT ( 'NONE',  ( 67.34521997529867576, 314.8592298662555322, 4.000000000000003553 ) ) ;
#19461=EDGE_LOOP ( 'NONE', ( #2356, #19884, #7149, #11798 ) ) ;
#19467=ORIENTED_EDGE ( 'NONE', *, *, #15712, .T. ) ;
#19468=ORIENTED_EDGE ( 'NONE', *, *, #8443, .T. ) ;
#19490=ORIENTED_EDGE ( 'NONE', *, *, #16914, .T. ) ;
#19492=ORIENTED_EDGE ( 'NONE', *, *, #5294, .T. ) ;
#19503=CARTESIAN_POINT ( 'NONE',  ( 147.5268905834513475, 193.0332408774651185, 272.0939500981630204 ) ) ;
#19520=FILL_AREA_STYLE_COLOUR ( '', #6420 ) ;
#19524=DIRECTION ( 'NONE',  ( 0.3450121214752274179, -0.9385982292947088190, 7.395570986446985676E-32 ) ) ;
#19551=CARTESIAN_POINT ( 'NONE',  ( 67.34521997529867576, 314.8592298662555322, -4.000000000000002665 ) ) ;
#19556=PRODUCT_CONTEXT ( 'NONE', #6034, 'mechanical' ) ;
#19584=SHAPE_REPRESENTATION_RELATIONSHIP ( 'NONE' , 'NONE' ,  #17468, #586 ) ;
#19605=CIRCLE ( 'NONE', #12558, 10.00000000000000888 ) ;
#19614=CARTESIAN_POINT ( 'NONE',  ( 84.42064422693164261, 282.0082918409407284, 4.000000000000003553 ) ) ;
#19618=VECTOR ( 'NONE', #11594, 1000.000000000000227 ) ;
#19619=DIRECTION ( 'NONE',  ( -0.000000000000000000, -0.000000000000000000, -1.000000000000000000 ) ) ;
#19634=( LENGTH_UNIT ( ) NAMED_UNIT ( * ) SI_UNIT ( .MILLI., .METRE. ) );
#19637=PLANE ( 'NONE',  #15377 ) ;
#19656=DIRECTION ( 'NONE',  ( 1.000000000000000000, 0.000000000000000000, 0.000000000000000000 ) ) ;
#19714=ORIENTED_EDGE ( 'NONE', *, *, #16774, .F. ) ;
#19772=VERTEX_POINT ( 'NONE', #3822 ) ;
#19787=VECTOR ( 'NONE', #19246, 1000.000000000000000 ) ;
#19801=ORIENTED_EDGE ( 'NONE', *, *, #2682, .T. ) ;
#19827=DIRECTION ( 'NONE',  ( 1.648795714028702312E-16, 6.060681657195960733E-17, 1.000000000000000000 ) ) ;
#19860=DIRECTION ( 'NONE',  ( -1.000000000000000000, 0.000000000000000000, 0.000000000000000000 ) ) ;
#19884=ORIENTED_EDGE ( 'NONE', *, *, #7644, .T. ) ;
#19922=CARTESIAN_POINT ( 'NONE',  ( 163.4517194221884040, 198.8869265230379995, -5.999999999999976019 ) ) ;
#19930=EDGE_CURVE ( 'NONE', #7143, #20168, #8620, .T. ) ;
#19950=AXIS2_PLACEMENT_3D ( 'NONE', #19614, #9378, #14214 ) ;
#19955=DIRECTION ( 'NONE',  ( -0.3450121214752278065, 0.9385982292947087080, -0.000000000000000000 ) ) ;
#19966=VERTEX_POINT ( 'NONE', #17722 ) ;
#20000=LINE ( 'NONE', #4665, #3940 ) ;
#20006=EDGE_LOOP ( 'NONE', ( #10615, #686, #16040, #21080 ) ) ;
#20039=ADVANCED_FACE ( 'NONE', ( #2233, #20542 ), #18993, .T. ) ;
#20070=DIRECTION ( 'NONE',  ( -1.000000000000000000, 0.000000000000000000, 0.000000000000000000 ) ) ;
#20073=LINE ( 'NONE', #4959, #18086 ) ;
#20084=CARTESIAN_POINT ( 'NONE',  ( 93.25569916848381524, 126.0916958004080755, -19.99999999999997868 ) ) ;
#20087=VERTEX_POINT ( 'NONE', #12667 ) ;
#20090=EDGE_LOOP ( 'NONE', ( #14148, #16369, #7773, #18132 ) ) ;
#20121=DIRECTION ( 'NONE',  ( 0.9385982292947088190, 0.3450121214752278620, -0.000000000000000000 ) ) ;
#20124=FACE_OUTER_BOUND ( 'NONE', #20006, .T. ) ;
#20143=AXIS2_PLACEMENT_3D ( 'NONE', #11748, #16924, #6913 ) ;
#20166=ADVANCED_FACE ( 'NONE', ( #12996 ), #12773, .F. ) ;
#20168=VERTEX_POINT ( 'NONE', #984 ) ;
#20241=AXIS2_PLACEMENT_3D ( 'NONE', #16170, #2731, #12655 ) ;
#20288=LINE ( 'NONE', #4177, #9578 ) ;
#20314=AXIS2_PLACEMENT_3D ( 'NONE', #20844, #9493, #5736 ) ;
#20328=CARTESIAN_POINT ( 'NONE',  ( 79.42064422693164261, 282.0082918409407284, -4.000000000000002665 ) ) ;
#20330=VECTOR ( 'NONE', #20519, 1000.000000000000000 ) ;
#20344=CIRCLE ( 'NONE', #10837, 5.000000000000004441 ) ;
#20347=PLANE ( 'NONE',  #17139 ) ;
#20374=EDGE_LOOP ( 'NONE', ( #21432, #19714, #9721, #10065 ) ) ;
#20377=CARTESIAN_POINT ( 'NONE',  ( 131.8222645499855901, 267.5435007770738025, -6.999999999999995559 ) ) ;
#20401=ORIENTED_EDGE ( 'NONE', *, *, #3541, .F. ) ;
#20404=EDGE_CURVE ( 'NONE', #2626, #9805, #7826, .T. ) ;
#20437=CLOSED_SHELL ( 'NONE', ( #241, #2998, #763, #5953, #18936, #21306, #10722, #13266, #1642, #2047, #15664, #12010, #2875, #13677, #2275, #20699, #12854, #1335, #10348, #20039, #11134, #19305, #8257, #18103 ) ) ;
#20439=PLANE ( 'NONE',  #6048 ) ;
#20451=ORIENTED_EDGE ( 'NONE', *, *, #1506, .F. ) ;
#20461=CARTESIAN_POINT ( 'NONE',  ( 137.5268905834513191, 193.0332408774651185, -19.99999999999997868 ) ) ;
#20467=CARTESIAN_POINT ( 'NONE',  ( 24.43941541943582862, 313.3049502139530205, 272.0939500981630204 ) ) ;
#20474=DIRECTION ( 'NONE',  ( -0.000000000000000000, -0.000000000000000000, -1.000000000000000000 ) ) ;
#20519=DIRECTION ( 'NONE',  ( -0.000000000000000000, -0.000000000000000000, -1.000000000000000000 ) ) ;
#20527=EDGE_CURVE ( 'NONE', #19772, #17982, #10133, .T. ) ;
#20531=ORIENTED_EDGE ( 'NONE', *, *, #14159, .F. ) ;
#20542=FACE_OUTER_BOUND ( 'NONE', #2349, .T. ) ;
#20560=DIRECTION ( 'NONE',  ( -0.000000000000000000, -0.000000000000000000, -1.000000000000000000 ) ) ;
#20563=EDGE_CURVE ( 'NONE', #21618, #8176, #13354, .T. ) ;
#20590=ORIENTED_EDGE ( 'NONE', *, *, #11064, .T. ) ;
#20657=LINE ( 'NONE', #3475, #14347 ) ;
#20660=VECTOR ( 'NONE', #9535, 1000.000000000000000 ) ;
#20674=AXIS2_PLACEMENT_3D ( 'NONE', #2213, #20121, #7403 ) ;
#20677=FACE_OUTER_BOUND ( 'NONE', #20090, .T. ) ;
#20699=ADVANCED_FACE ( 'NONE', ( #10890, #4160, #20809, #9241 ), #5700, .T. ) ;
#20773=LINE ( 'NONE', #19012, #12035 ) ;
#20809=FACE_BOUND ( 'NONE', #4015, .T. ) ;
#20829=EDGE_CURVE ( 'NONE', #15960, #20168, #16267, .T. ) ;
#20844=CARTESIAN_POINT ( 'NONE',  ( 72.34521997529867576, 314.8592298662555322, -4.000000000000003553 ) ) ;
#20848=CARTESIAN_POINT ( 'NONE',  ( 96.62434152388762243, 220.7958015105191976, -5.999999999999976019 ) ) ;
#20857=VERTEX_POINT ( 'NONE', #1173 ) ;
#20911=VECTOR ( 'NONE', #17689, 1000.000000000000000 ) ;
#20930=EDGE_CURVE ( 'NONE', #1138, #17533, #9671, .T. ) ;
#20952=DIRECTION ( 'NONE',  ( 0.000000000000000000, 0.000000000000000000, 1.000000000000000000 ) ) ;
#20995=ORIENTED_EDGE ( 'NONE', *, *, #20829, .F. ) ;
#21003=DIRECTION ( 'NONE',  ( -0.5250363069212118372, 0.8510798296367592108, 0.000000000000000000 ) ) ;
#21019=EDGE_LOOP ( 'NONE', ( #21108, #13321 ) ) ;
#21020=LINE ( 'NONE', #10770, #632 ) ;
#21055=ORIENTED_EDGE ( 'NONE', *, *, #13773, .F. ) ;
#21080=ORIENTED_EDGE ( 'NONE', *, *, #15000, .F. ) ;
#21086=CARTESIAN_POINT ( 'NONE',  ( 147.5268905834513475, 193.0332408774651185, -19.99999999999997868 ) ) ;
#21101=ORIENTED_EDGE ( 'NONE', *, *, #3369, .F. ) ;
#21103=AXIS2_PLACEMENT_3D ( 'NONE', #19363, #13962, #19046 ) ;
#21108=ORIENTED_EDGE ( 'NONE', *, *, #10803, .T. ) ;
#21167=DIRECTION ( 'NONE',  ( 1.915514545828640458E-16, 7.041092946335503408E-17, 1.000000000000000000 ) ) ;
#21176=EDGE_LOOP ( 'NONE', ( #18192, #9971, #18960, #10131, #11800, #17637 ) ) ;
#21199=LINE ( 'NONE', #1461, #13440 ) ;
#21254=FACE_OUTER_BOUND ( 'NONE', #9944, .T. ) ;
#21288=ORIENTED_EDGE ( 'NONE', *, *, #17549, .F. ) ;
#21295=VERTEX_POINT ( 'NONE', #20461 ) ;
#21306=ADVANCED_FACE ( 'NONE', ( #3704 ), #12507, .F. ) ;
#21320=AXIS2_PLACEMENT_3D ( 'NONE', #17919, #7914, #2828 ) ;
#21355=CARTESIAN_POINT ( 'NONE',  ( 163.4517194221884040, 198.8869265230379995, -19.99999999999997868 ) ) ;
#21384=FACE_OUTER_BOUND ( 'NONE', #3126, .T. ) ;
#21415=CARTESIAN_POINT ( 'NONE',  ( -56.84366818088135176, 789.5005544000622422, -19.99999999999997868 ) ) ;
#21428=DIRECTION ( 'NONE',  ( 0.3450121214752276400, -0.9385982292947087080, -0.000000000000000000 ) ) ;
#21432=ORIENTED_EDGE ( 'NONE', *, *, #11333, .T. ) ;
#21450=DIRECTION ( 'NONE',  ( -0.9385982292947088190, -0.3450121214752278620, 0.000000000000000000 ) ) ;
#21461=DIRECTION ( 'NONE',  ( 0.9385982292947087080, 0.3450121214752278620, -1.836742322155470738E-16 ) ) ;
#21469=EDGE_CURVE ( 'NONE', #17427, #1334, #17223, .T. ) ;
#21483=ORIENTED_EDGE ( 'NONE', *, *, #15154, .T. ) ;
#21488=DIRECTION ( 'NONE',  ( 1.000000000000000000, 0.000000000000000000, -1.648795714028702312E-16 ) ) ;
#21519=EDGE_LOOP ( 'NONE', ( #13558, #1165, #18665, #7330 ) ) ;
#21542=ORIENTED_EDGE ( 'NONE', *, *, #1506, .T. ) ;
#21608=PLANE ( 'NONE',  #17457 ) ;
#21618=VERTEX_POINT ( 'NONE', #19551 ) ;
#21637=LINE ( 'NONE', #13249, #17445 ) ;
#21664=CARTESIAN_POINT ( 'NONE',  ( 101.6431471920911207, 239.2647937927896464, 4.000000000000021316 ) ) ;
#21667=DIRECTION ( 'NONE',  ( -1.000000000000000000, 0.000000000000000000, 0.000000000000000000 ) ) ;
#21675=AXIS2_PLACEMENT_3D ( 'NONE', #15513, #13957, #15612 ) ;
#21704=DIRECTION ( 'NONE',  ( -0.8835682276357670339, -0.4683024526015100442, 0.000000000000000000 ) ) ;
#21732=VERTEX_POINT ( 'NONE', #13163 ) ;
#21754=ORIENTED_EDGE ( 'NONE', *, *, #18056, .T. ) ;
#21764=ORIENTED_EDGE ( 'NONE', *, *, #11064, .F. ) ;
#21765=AXIS2_PLACEMENT_3D ( 'NONE', #670, #455, #12242 ) ;
#21767=DIRECTION ( 'NONE',  ( -0.3450121214752276400, 0.9385982292947087080, 0.000000000000000000 ) ) ;
#21811=VECTOR ( 'NONE', #16618, 1000.000000000000000 ) ;
#21817=DIRECTION ( 'NONE',  ( 1.000000000000000000, 0.000000000000000000, -1.734723475976805615E-16 ) ) ;
ENDSEC;
END-ISO-10303-21;
